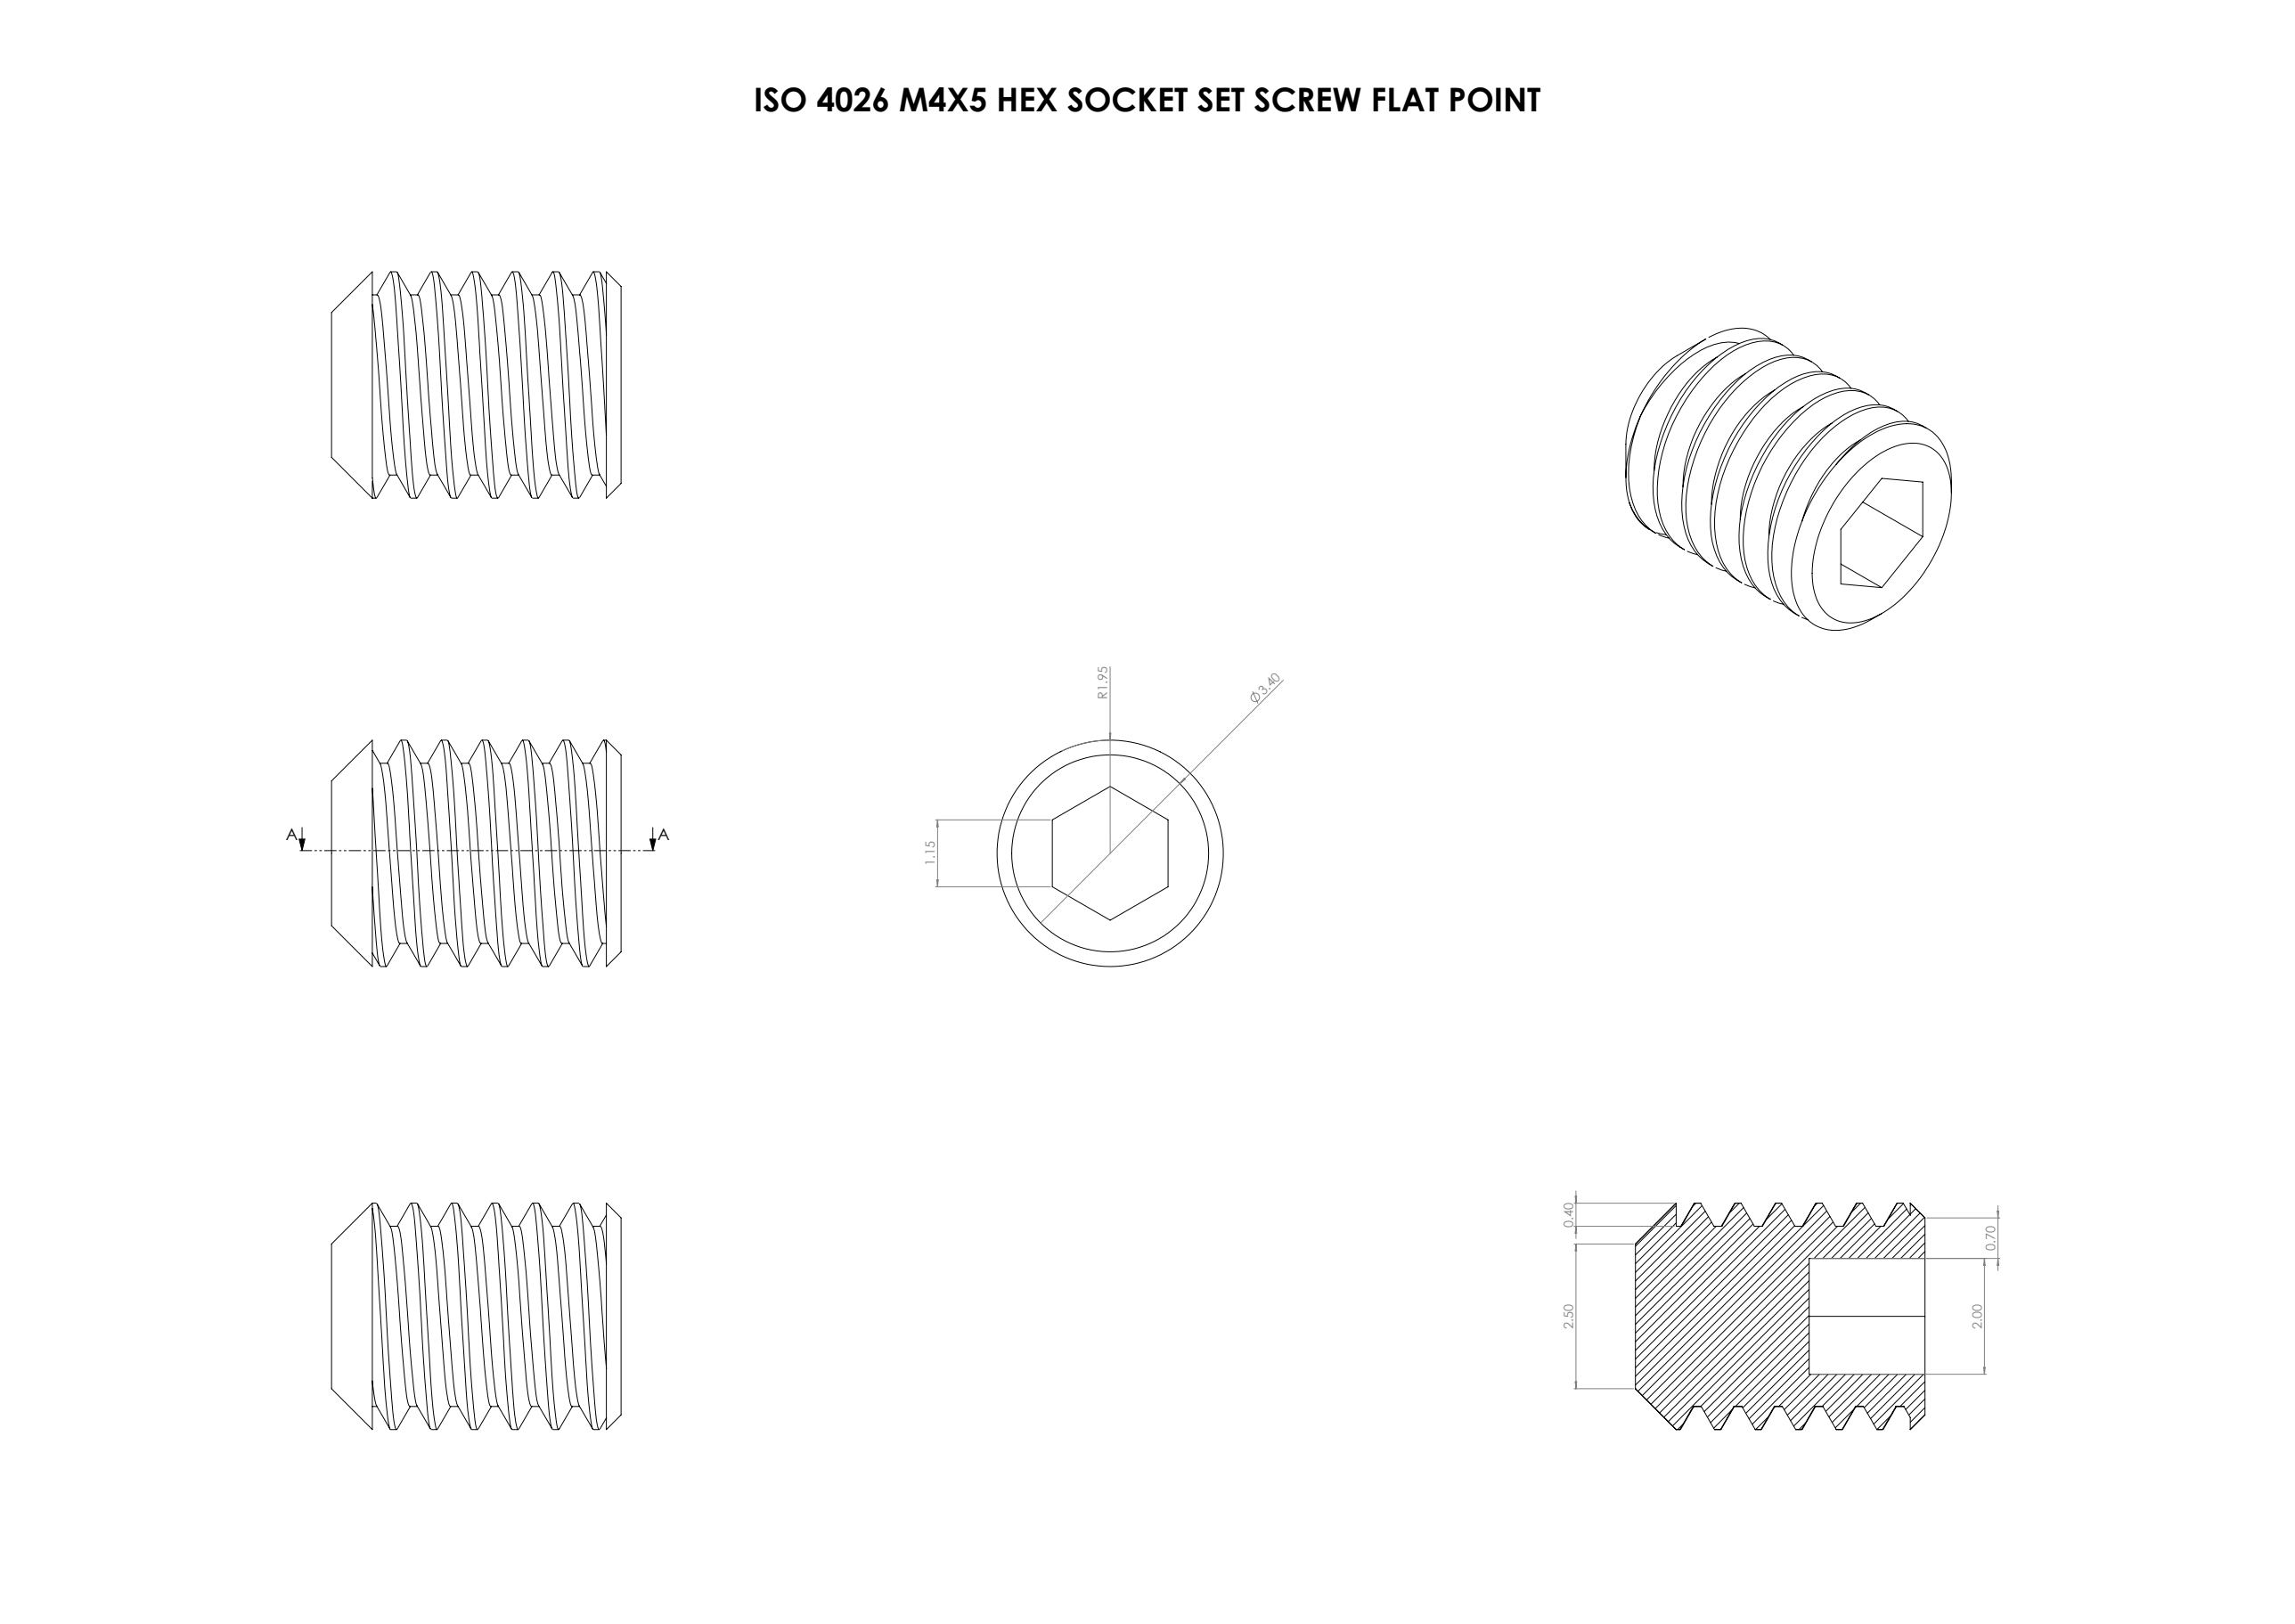
ISO-10303-21;
HEADER;
/* Generated by software containing ST-Developer
 * from STEP Tools, Inc. (www.steptools.com) 
 */

FILE_DESCRIPTION(
/* description */ (''),
/* implementation_level */ '2;1');

FILE_NAME(
/* name */ 
'08_ISO_4026_M4x5_Hex_Socket_Set_Screw_Flat_Point.step',
/* time_stamp */ '2026-10-22T00:21:42-07:00',
/* author */ (''),
/* organization */ (''),
/* preprocessor_version */ 'ST-DEVELOPER v20.2',
/* originating_system */ 'Autodesk Translation Framework v15.15.0.0',
/* authorisation */ '');

FILE_SCHEMA (('AUTOMOTIVE_DESIGN { 1 0 10303 214 3 1 1 }'));
ENDSEC;

DATA;
#10=MECHANICAL_DESIGN_GEOMETRIC_PRESENTATION_REPRESENTATION('',(#212),#31638);
#190=SHAPE_REPRESENTATION_RELATIONSHIP('SRR','None',#31712,#201);
#201=ADVANCED_BREP_SHAPE_REPRESENTATION('',(#223),#31634);
#212=STYLED_ITEM('',(#31837),#223);
#223=MANIFOLD_SOLID_BREP('Set screw',#12487);
#293=CYLINDRICAL_SURFACE('',#13137,0.1954);
#294=CYLINDRICAL_SURFACE('',#13139,0.1954);
#295=CYLINDRICAL_SURFACE('',#13140,0.1954);
#296=CYLINDRICAL_SURFACE('',#13141,0.1954);
#297=CYLINDRICAL_SURFACE('',#13142,0.1954);
#298=CYLINDRICAL_SURFACE('',#13143,0.1954);
#299=CYLINDRICAL_SURFACE('',#13144,0.15555);
#300=CYLINDRICAL_SURFACE('',#13146,0.15555);
#301=CYLINDRICAL_SURFACE('',#13148,0.15555);
#302=CYLINDRICAL_SURFACE('',#13149,0.15555);
#303=CYLINDRICAL_SURFACE('',#13150,0.15555);
#304=CYLINDRICAL_SURFACE('',#13151,0.15555);
#305=CYLINDRICAL_SURFACE('',#13159,0.15555);
#306=CYLINDRICAL_SURFACE('',#13170,0.1954);
#435=CONICAL_SURFACE('',#13169,0.185,0.785398163397445);
#436=CONICAL_SURFACE('',#13172,0.1625,0.785398163397447);
#1015=B_SPLINE_CURVE_WITH_KNOTS('',3,(#25849,#25850,#25851,#25852,#25853,
#25854,#25855,#25856,#25857,#25858),.UNSPECIFIED.,.F.,.F.,(4,3,3,4),(-4.09254174883833,
-3.93292792746001,-2.94969594559501,-2.0651401332781),.UNSPECIFIED.);
#1016=B_SPLINE_CURVE_WITH_KNOTS('',3,(#25861,#25862,#25863,#25864,#25865,
#25866,#25867),.UNSPECIFIED.,.F.,.F.,(4,3,4),(0.,0.983231981865002,1.11419103802958),
 .UNSPECIFIED.);
#1017=B_SPLINE_CURVE_WITH_KNOTS('',3,(#25872,#25873,#25874,#25875,#25876,
#25877,#25878,#25879,#25880,#25881,#25882,#25883,#25884,#25885,#25886,#25887,
#25888,#25889,#25890,#25891,#25892,#25893),.UNSPECIFIED.,.F.,.F.,(4,3,3,
3,3,3,3,4),(-10.3757270560179,-9.83231981865002,-8.84908783678502,-7.86585585492002,
-6.88262387305502,-5.89939189119002,-4.91615990932501,-4.09254174883833),
 .UNSPECIFIED.);
#1018=B_SPLINE_CURVE_WITH_KNOTS('',3,(#25894,#25895,#25896,#25897,#25898,
#25899,#25900,#25901,#25902,#25903,#25904,#25905,#25906,#25907,#25908,#25909,
#25910,#25911,#25912,#25913,#25914,#25915),.UNSPECIFIED.,.F.,.F.,(4,3,3,
3,3,3,3,4),(1.11419103802958,1.96646396373,2.94969594559501,3.93292792746001,
4.91615990932501,5.89939189119001,6.88262387305501,7.39737634520916),
 .UNSPECIFIED.);
#1019=B_SPLINE_CURVE_WITH_KNOTS('',3,(#25920,#25921,#25922,#25923,#25924,
#25925,#25926,#25927,#25928,#25929,#25930,#25931,#25932,#25933,#25934,#25935,
#25936,#25937,#25938,#25939,#25940,#25941),.UNSPECIFIED.,.F.,.F.,(4,3,3,
3,3,3,3,4),(-16.6589123631975,-15.73171170984,-14.748479727975,-13.76524774611,
-12.782015764245,-11.79878378238,-10.815551800515,-10.3757270560179),
 .UNSPECIFIED.);
#1020=B_SPLINE_CURVE_WITH_KNOTS('',3,(#25942,#25943,#25944,#25945,#25946,
#25947,#25948,#25949,#25950,#25951,#25952,#25953,#25954,#25955,#25956,#25957,
#25958,#25959,#25960,#25961,#25962,#25963),.UNSPECIFIED.,.F.,.F.,(4,3,3,
3,3,3,3,4),(7.39737634520916,7.86585585492002,8.84908783678502,9.83231981865002,
10.815551800515,11.79878378238,12.782015764245,13.6805616523888),
 .UNSPECIFIED.);
#1021=B_SPLINE_CURVE_WITH_KNOTS('',3,(#25968,#25969,#25970,#25971,#25972,
#25973,#25974,#25975,#25976,#25977,#25978,#25979,#25980,#25981,#25982,#25983,
#25984,#25985,#25986,#25987,#25988,#25989,#25990,#25991,#25992),
 .UNSPECIFIED.,.F.,.F.,(4,3,3,3,3,3,3,3,4),(-22.9420976703771,-22.6143355828951,
-21.6311036010301,-20.647871619165,-19.6646396373,-18.681407655435,-17.69817567357,
-16.714943691705,-16.6589123631975),.UNSPECIFIED.);
#1022=B_SPLINE_CURVE_WITH_KNOTS('',3,(#25993,#25994,#25995,#25996,#25997,
#25998,#25999,#26000,#26001,#26002,#26003,#26004,#26005,#26006,#26007,#26008,
#26009,#26010,#26011,#26012,#26013,#26014,#26015,#26016,#26017),
 .UNSPECIFIED.,.F.,.F.,(4,3,3,3,3,3,3,3,4),(13.6805616523888,13.76524774611,
14.748479727975,15.73171170984,16.714943691705,17.69817567357,18.681407655435,
19.6646396373,19.9637469595683),.UNSPECIFIED.);
#1023=B_SPLINE_CURVE_WITH_KNOTS('',3,(#26022,#26023,#26024,#26025,#26026,
#26027,#26028,#26029,#26030,#26031,#26032,#26033,#26034,#26035,#26036,#26037,
#26038,#26039,#26040,#26041,#26042,#26043),.UNSPECIFIED.,.F.,.F.,(4,3,3,
3,3,3,3,4),(-29.2252829775567,-28.5137274740851,-27.5304954922201,-26.5472635103551,
-25.5640315284901,-24.5807995466251,-23.5975675647601,-22.9420976703771),
 .UNSPECIFIED.);
#1024=B_SPLINE_CURVE_WITH_KNOTS('',3,(#26044,#26045,#26046,#26047,#26048,
#26049,#26050,#26051,#26052,#26053,#26054,#26055,#26056,#26057,#26058,#26059,
#26060,#26061,#26062,#26063,#26064,#26065),.UNSPECIFIED.,.F.,.F.,(4,3,3,
3,3,3,3,4),(19.9637469595683,20.647871619165,21.63110360103,22.614335582895,
23.59756756476,24.580799546625,25.5640315284901,26.2469322667479),
 .UNSPECIFIED.);
#1025=B_SPLINE_CURVE_WITH_KNOTS('',3,(#26070,#26071,#26072,#26073,#26074,
#26075,#26076,#26077,#26078,#26079,#26080,#26081,#26082,#26083,#26084,#26085,
#26086,#26087,#26088,#26089,#26090,#26091,#26092,#26093,#26094),
 .UNSPECIFIED.,.F.,.F.,(4,3,3,3,3,3,3,3,4),(-35.5084682847363,-35.3963513471401,
-34.4131193652751,-33.4298873834101,-32.4466554015451,-31.4634234196801,
-30.4801914378151,-29.4969594559501,-29.2252829775567),.UNSPECIFIED.);
#1026=B_SPLINE_CURVE_WITH_KNOTS('',3,(#26095,#26096,#26097,#26098,#26099,
#26100,#26101,#26102,#26103,#26104,#26105,#26106,#26107,#26108,#26109,#26110,
#26111,#26112,#26113,#26114,#26115,#26116,#26117,#26118,#26119),
 .UNSPECIFIED.,.F.,.F.,(4,3,3,3,3,3,3,3,4),(26.2469322667479,26.547263510355,
27.5304954922201,28.5137274740851,29.4969594559501,30.4801914378151,31.4634234196801,
32.4466554015451,32.5301175739275),.UNSPECIFIED.);
#1027=B_SPLINE_CURVE_WITH_KNOTS('',3,(#26125,#26126,#26127,#26128),
 .UNSPECIFIED.,.F.,.F.,(4,4),(47.1238898038469,47.8963286785676),
 .UNSPECIFIED.);
#1028=B_SPLINE_CURVE_WITH_KNOTS('',3,(#26134,#26135,#26136,#26137,#26138,
#26139,#26140,#26141,#26142,#26143,#26144),.UNSPECIFIED.,.F.,.F.,(4,1,1,
1,1,1,1,1,4),(40.8407044966673,41.1123809750607,42.0956129569257,43.0788449387907,
44.0620769206557,45.0453089025207,46.0285408843857,47.0117728662507,47.1238898038469),
 .UNSPECIFIED.);
#1029=B_SPLINE_CURVE_WITH_KNOTS('',3,(#26147,#26148,#26149,#26150,#26151,
#26152,#26153,#26154,#26155),.UNSPECIFIED.,.F.,.F.,(4,1,1,1,1,1,4),(40.8407044966673,
41.7404743061498,42.7237062880148,43.7069382698798,44.6901702517448,45.6734022336098,
46.6566342154749),.UNSPECIFIED.);
#1030=B_SPLINE_CURVE_WITH_KNOTS('',3,(#26160,#26161,#26162,#26163,#26164,
#26165,#26166,#26167,#26168,#26169),.UNSPECIFIED.,.F.,.F.,(4,1,1,1,1,1,
1,4),(34.5575191894877,35.2129890838707,36.1962210657357,37.1794530476007,
38.1626850294657,39.1459170113307,40.1291489931957,40.8407044966673),
 .UNSPECIFIED.);
#1031=B_SPLINE_CURVE_WITH_KNOTS('',3,(#26170,#26171,#26172,#26173,#26174,
#26175,#26176,#26177,#26178,#26179,#26180),.UNSPECIFIED.,.F.,.F.,(4,1,1,
1,1,1,1,1,4),(34.5575191894877,34.8578504330948,35.8410824149598,36.8243143968248,
37.8075463786898,38.7907783605548,39.7740103424198,40.7572423242848,40.8407044966673),
 .UNSPECIFIED.);
#1032=B_SPLINE_CURVE_WITH_KNOTS('',3,(#26185,#26186,#26187,#26188,#26189,
#26190,#26191,#26192,#26193,#26194,#26195),.UNSPECIFIED.,.F.,.F.,(4,1,1,
1,1,1,1,1,4),(28.2743338823081,28.3303652108157,29.3135971926807,30.2968291745457,
31.2800611564107,32.2632931382757,33.2465251201407,34.2297571020057,34.5575191894877),
 .UNSPECIFIED.);
#1033=B_SPLINE_CURVE_WITH_KNOTS('',3,(#26196,#26197,#26198,#26199,#26200,
#26201,#26202,#26203,#26204,#26205),.UNSPECIFIED.,.F.,.F.,(4,1,1,1,1,1,
1,4),(28.2743338823081,28.9584585419048,29.9416905237698,30.9249225056348,
31.9081544874998,32.8913864693648,33.8746184512298,34.5575191894877),
 .UNSPECIFIED.);
#1034=B_SPLINE_CURVE_WITH_KNOTS('',3,(#26210,#26211,#26212,#26213,#26214,
#26215,#26216,#26217,#26218,#26219),.UNSPECIFIED.,.F.,.F.,(4,1,1,1,1,1,
1,4),(21.9911485751285,22.4309733196257,23.4142053014907,24.3974372833557,
25.3806692652207,26.3639012470857,27.3471332289507,28.2743338823081),
 .UNSPECIFIED.);
#1035=B_SPLINE_CURVE_WITH_KNOTS('',3,(#26220,#26221,#26222,#26223,#26224,
#26225,#26226,#26227,#26228,#26229,#26230),.UNSPECIFIED.,.F.,.F.,(4,1,1,
1,1,1,1,1,4),(21.9911485751285,22.0758346688498,23.0590666507148,24.0422986325798,
25.0255306144448,26.0087625963098,26.9919945781748,27.9752265600398,28.2743338823081),
 .UNSPECIFIED.);
#1036=B_SPLINE_CURVE_WITH_KNOTS('',3,(#26235,#26236,#26237,#26238,#26239,
#26240,#26241,#26242,#26243,#26244),.UNSPECIFIED.,.F.,.F.,(4,1,1,1,1,1,
1,4),(15.707963267949,16.5315814284356,17.5148134103006,18.4980453921656,
19.4812773740306,20.4645093558957,21.4477413377607,21.9911485751285),
 .UNSPECIFIED.);
#1037=B_SPLINE_CURVE_WITH_KNOTS('',3,(#26245,#26246,#26247,#26248,#26249,
#26250,#26251,#26252,#26253,#26254),.UNSPECIFIED.,.F.,.F.,(4,1,1,1,1,1,
1,4),(15.707963267949,16.1764427776598,17.1596747595248,18.1429067413898,
19.1261387232548,20.1093707051198,21.0926026869848,21.9911485751285),
 .UNSPECIFIED.);
#1038=B_SPLINE_CURVE_WITH_KNOTS('',3,(#26257,#26258,#26259,#26260,#26261,
#26262,#26263,#26264,#26265,#26266,#26267,#26268,#26269,#26270,#26271,#26272,
#26273,#26274,#26275,#26276,#26277,#26278,#26279,#26280,#26281,#26282,#26283,
#26284,#26285,#26286,#26287,#26288,#26289,#26290,#26291,#26292,#26293,#26294,
#26295,#26296,#26297,#26298,#26299,#26300,#26301,#26302,#26303,#26304,#26305,
#26306,#26307,#26308),.UNSPECIFIED.,.F.,.F.,(4,3,3,3,3,3,3,3,3,3,3,3,3,
3,3,3,3,4),(-0.366397579005844,-0.350753953906653,-0.330463017686532,-0.315435531128199,
-0.287643881494464,-0.272924732924834,-0.237814891323476,-0.221795460451242,
-0.207726041133023,-0.184571159408416,-0.160894855415823,-0.147419681563097,
-0.13576580392061,-0.101824352940458,-0.0769585672558313,-0.0671142413070353,
-0.0286195295740189,0.),.UNSPECIFIED.);
#1039=B_SPLINE_CURVE_WITH_KNOTS('',3,(#26313,#26314,#26315,#26316,#26317,
#26318,#26319,#26320,#26321,#26322,#26323,#26324,#26325,#26326,#26327,#26328,
#26329,#26330,#26331,#26332,#26333,#26334,#26335,#26336,#26337,#26338,#26339,
#26340,#26341,#26342,#26343,#26344,#26345,#26346,#26347,#26348,#26349,#26350,
#26351,#26352,#26353,#26354,#26355,#26356,#26357,#26358,#26359,#26360,#26361,
#26362,#26363,#26364,#26365,#26366,#26367),.UNSPECIFIED.,.F.,.F.,(4,3,3,
3,3,3,3,3,3,3,3,3,3,3,3,3,3,3,4),(-0.364629307890667,-0.345405509511423,
-0.316109491299348,-0.303964239439482,-0.281709554317525,-0.264921543558191,
-0.252375276770721,-0.215944087132777,-0.198753901855764,-0.18596810420685,
-0.163689794923203,-0.143278793185558,-0.127728424538677,-0.117434610457182,
-0.0880759578428862,-0.0702652452140735,-0.0601818930641948,-0.0277041096514565,
0.),.UNSPECIFIED.);
#1040=B_SPLINE_CURVE_WITH_KNOTS('',3,(#26536,#26537,#26538,#26539,#26540,
#26541,#26542,#26543,#26544,#26545,#26546,#26547,#26548),.UNSPECIFIED.,
 .F.,.F.,(4,3,3,3,4),(32.5301175739275,33.4298873834101,34.4131193652751,
35.3963513471401,36.280907159457),.UNSPECIFIED.);
#1041=B_SPLINE_CURVE_WITH_KNOTS('',3,(#26550,#26551,#26552,#26553,#26554,
#26555,#26556,#26557,#26558,#26559,#26560,#26561,#26562,#26563,#26564,#26565,
#26566,#26567,#26568,#26569,#26570,#26571,#26572,#26573,#26574,#26575,#26576,
#26577,#26578,#26579,#26580,#26581,#26582,#26583,#26584,#26585,#26586,#26587,
#26588,#26589,#26590,#26591,#26592,#26593,#26594,#26595,#26596,#26597,#26598,
#26599,#26600,#26601),.UNSPECIFIED.,.F.,.F.,(4,3,3,3,3,3,3,3,3,3,3,3,3,
3,3,3,3,4),(-0.366397579005851,-0.350753953906661,-0.330463024735024,-0.315435543259483,
-0.287644877982493,-0.272925011059114,-0.237815179368718,-0.221795848896316,
-0.207726060922694,-0.184571159408424,-0.160894850055595,-0.147419600331868,
-0.135765787605129,-0.101824340703847,-0.0769585196865098,-0.0671141722159687,
-0.0286194368321035,0.),.UNSPECIFIED.);
#1042=B_SPLINE_CURVE_WITH_KNOTS('',3,(#26602,#26603,#26604,#26605,#26606,
#26607,#26608,#26609,#26610),.UNSPECIFIED.,.F.,.F.,(4,1,1,1,1,1,4),(10.3757270560179,
11.2602828683348,12.2435148501998,13.2267468320648,14.2099788139298,15.1932107957948,
15.707963267949),.UNSPECIFIED.);
#1043=B_SPLINE_CURVE_WITH_KNOTS('',3,(#26616,#26617,#26618,#26619,#26620,
#26621,#26622,#26623,#26624,#26625,#26626,#26627,#26628,#26629,#26630,#26631,
#26632,#26633,#26634,#26635,#26636,#26637,#26638,#26639,#26640,#26641,#26642,
#26643,#26644,#26645,#26646,#26647,#26648,#26649,#26650,#26651,#26652,#26653,
#26654,#26655,#26656,#26657,#26658,#26659,#26660,#26661,#26662,#26663,#26664,
#26665,#26666,#26667,#26668,#26669,#26670),.UNSPECIFIED.,.F.,.F.,(4,3,3,
3,3,3,3,3,3,3,3,3,3,3,3,3,3,3,4),(-0.364629307890684,-0.345405509511438,
-0.316109466616483,-0.303964180518109,-0.28170938055002,-0.264921036000774,
-0.252375151029453,-0.215943930999405,-0.198753706254068,-0.185968021399695,
-0.163689794923211,-0.143278681804942,-0.127728193637607,-0.117434275921994,
-0.0880757069414953,-0.070264744543059,-0.0601814248546799,-0.0277037327266843,
0.),.UNSPECIFIED.);
#1044=B_SPLINE_CURVE_WITH_KNOTS('',3,(#26673,#26674,#26675,#26676,#26677,
#26678,#26679,#26680),.UNSPECIFIED.,.F.,.F.,(4,1,1,1,1,4),(11.6154215191106,
12.5986535009756,13.5818854828406,14.5651174647056,15.5483494465706,15.707963267949),
 .UNSPECIFIED.);
#1045=B_SPLINE_CURVE_WITH_KNOTS('',3,(#26849,#26850,#26851,#26852,#26853,
#26854,#26855,#26856,#26857,#26858),.UNSPECIFIED.,.F.,.F.,(4,3,3,4),(-38.3460472927351,
-37.3628153108701,-36.3795833290051,-35.5084682847363),.UNSPECIFIED.);
#1330=B_SPLINE_SURFACE_WITH_KNOTS('',3,3,((#26368,#26369,#26370,#26371,
#26372,#26373,#26374,#26375,#26376,#26377,#26378,#26379,#26380,#26381,#26382,
#26383,#26384,#26385,#26386,#26387,#26388,#26389,#26390,#26391,#26392,#26393,
#26394,#26395,#26396,#26397,#26398,#26399,#26400,#26401,#26402,#26403,#26404,
#26405,#26406,#26407,#26408,#26409),(#26410,#26411,#26412,#26413,#26414,
#26415,#26416,#26417,#26418,#26419,#26420,#26421,#26422,#26423,#26424,#26425,
#26426,#26427,#26428,#26429,#26430,#26431,#26432,#26433,#26434,#26435,#26436,
#26437,#26438,#26439,#26440,#26441,#26442,#26443,#26444,#26445,#26446,#26447,
#26448,#26449,#26450,#26451),(#26452,#26453,#26454,#26455,#26456,#26457,
#26458,#26459,#26460,#26461,#26462,#26463,#26464,#26465,#26466,#26467,#26468,
#26469,#26470,#26471,#26472,#26473,#26474,#26475,#26476,#26477,#26478,#26479,
#26480,#26481,#26482,#26483,#26484,#26485,#26486,#26487,#26488,#26489,#26490,
#26491,#26492,#26493),(#26494,#26495,#26496,#26497,#26498,#26499,#26500,
#26501,#26502,#26503,#26504,#26505,#26506,#26507,#26508,#26509,#26510,#26511,
#26512,#26513,#26514,#26515,#26516,#26517,#26518,#26519,#26520,#26521,#26522,
#26523,#26524,#26525,#26526,#26527,#26528,#26529,#26530,#26531,#26532,#26533,
#26534,#26535)),.UNSPECIFIED.,.F.,.F.,.F.,(4,4),(4,1,1,1,1,1,1,1,1,1,1,
1,1,1,1,1,1,1,1,1,1,1,1,1,1,1,1,1,1,1,1,1,1,1,1,1,1,1,1,4),(0.,0.0460148164544131),
(8.31058692273978,9.29381890460478,10.2770508864698,11.2602828683348,12.2435148501998,
13.2267468320648,14.2099788139298,15.1932107957948,16.1764427776598,17.1596747595248,
18.1429067413898,19.1261387232548,20.1093707051198,21.0926026869848,22.0758346688498,
23.0590666507148,24.0422986325798,25.0255306144448,26.0087625963098,26.9919945781748,
27.9752265600398,28.9584585419048,29.9416905237698,30.9249225056348,31.9081544874998,
32.8913864693648,33.8746184512298,34.8578504330948,35.8410824149598,36.8243143968248,
37.8075463786898,38.7907783605548,39.7740103424198,40.7572423242848,41.7404743061498,
42.7237062880148,43.7069382698798,44.6901702517448,45.6734022336098,46.6566342154749),
 .UNSPECIFIED.);
#1331=B_SPLINE_SURFACE_WITH_KNOTS('',3,3,((#26681,#26682,#26683,#26684,
#26685,#26686,#26687,#26688,#26689,#26690,#26691,#26692,#26693,#26694,#26695,
#26696,#26697,#26698,#26699,#26700,#26701,#26702,#26703,#26704,#26705,#26706,
#26707,#26708,#26709,#26710,#26711,#26712,#26713,#26714,#26715,#26716,#26717,
#26718,#26719,#26720,#26721,#26722),(#26723,#26724,#26725,#26726,#26727,
#26728,#26729,#26730,#26731,#26732,#26733,#26734,#26735,#26736,#26737,#26738,
#26739,#26740,#26741,#26742,#26743,#26744,#26745,#26746,#26747,#26748,#26749,
#26750,#26751,#26752,#26753,#26754,#26755,#26756,#26757,#26758,#26759,#26760,
#26761,#26762,#26763,#26764),(#26765,#26766,#26767,#26768,#26769,#26770,
#26771,#26772,#26773,#26774,#26775,#26776,#26777,#26778,#26779,#26780,#26781,
#26782,#26783,#26784,#26785,#26786,#26787,#26788,#26789,#26790,#26791,#26792,
#26793,#26794,#26795,#26796,#26797,#26798,#26799,#26800,#26801,#26802,#26803,
#26804,#26805,#26806),(#26807,#26808,#26809,#26810,#26811,#26812,#26813,
#26814,#26815,#26816,#26817,#26818,#26819,#26820,#26821,#26822,#26823,#26824,
#26825,#26826,#26827,#26828,#26829,#26830,#26831,#26832,#26833,#26834,#26835,
#26836,#26837,#26838,#26839,#26840,#26841,#26842,#26843,#26844,#26845,#26846,
#26847,#26848)),.UNSPECIFIED.,.F.,.F.,.F.,(4,4),(4,1,1,1,1,1,1,1,1,1,1,
1,1,1,1,1,1,1,1,1,1,1,1,1,1,1,1,1,1,1,1,1,1,1,1,1,1,1,1,4),(0.,0.0460148164544132),
(11.6154215191106,12.5986535009756,13.5818854828406,14.5651174647056,15.5483494465706,
16.5315814284356,17.5148134103006,18.4980453921656,19.4812773740306,20.4645093558957,
21.4477413377607,22.4309733196257,23.4142053014907,24.3974372833557,25.3806692652207,
26.3639012470857,27.3471332289507,28.3303652108157,29.3135971926807,30.2968291745457,
31.2800611564107,32.2632931382757,33.2465251201407,34.2297571020057,35.2129890838707,
36.1962210657357,37.1794530476007,38.1626850294657,39.1459170113307,40.1291489931957,
41.1123809750607,42.0956129569257,43.0788449387907,44.0620769206557,45.0453089025207,
46.0285408843857,47.0117728662507,47.9950048481157,48.9782368299807,49.9614688118457),
 .UNSPECIFIED.);
#1396=FACE_BOUND('',#2997,.T.);
#1657=CIRCLE('',#13138,0.1954);
#1658=CIRCLE('',#13145,0.15555);
#1659=CIRCLE('',#13147,0.15555);
#1660=CIRCLE('',#13153,0.1954);
#1661=CIRCLE('',#13154,0.1954);
#1662=CIRCLE('',#13156,0.1954);
#1663=CIRCLE('',#13157,0.1954);
#1664=CIRCLE('',#13158,0.15555);
#1665=CIRCLE('',#13168,0.17);
#1666=CIRCLE('',#13171,0.1954);
#1667=CIRCLE('',#13173,0.125);
#2222=FACE_OUTER_BOUND('',#2972,.T.);
#2223=FACE_OUTER_BOUND('',#2973,.T.);
#2224=FACE_OUTER_BOUND('',#2974,.T.);
#2225=FACE_OUTER_BOUND('',#2975,.T.);
#2226=FACE_OUTER_BOUND('',#2976,.T.);
#2227=FACE_OUTER_BOUND('',#2977,.T.);
#2228=FACE_OUTER_BOUND('',#2978,.T.);
#2229=FACE_OUTER_BOUND('',#2979,.T.);
#2230=FACE_OUTER_BOUND('',#2980,.T.);
#2231=FACE_OUTER_BOUND('',#2981,.T.);
#2232=FACE_OUTER_BOUND('',#2982,.T.);
#2233=FACE_OUTER_BOUND('',#2983,.T.);
#2234=FACE_OUTER_BOUND('',#2984,.T.);
#2235=FACE_OUTER_BOUND('',#2985,.T.);
#2236=FACE_OUTER_BOUND('',#2986,.T.);
#2237=FACE_OUTER_BOUND('',#2987,.T.);
#2238=FACE_OUTER_BOUND('',#2988,.T.);
#2239=FACE_OUTER_BOUND('',#2989,.T.);
#2240=FACE_OUTER_BOUND('',#2990,.T.);
#2241=FACE_OUTER_BOUND('',#2991,.T.);
#2242=FACE_OUTER_BOUND('',#2992,.T.);
#2243=FACE_OUTER_BOUND('',#2993,.T.);
#2244=FACE_OUTER_BOUND('',#2994,.T.);
#2245=FACE_OUTER_BOUND('',#2995,.T.);
#2246=FACE_OUTER_BOUND('',#2996,.T.);
#2247=FACE_OUTER_BOUND('',#2998,.T.);
#2248=FACE_OUTER_BOUND('',#2999,.T.);
#2249=FACE_OUTER_BOUND('',#3000,.T.);
#2250=FACE_OUTER_BOUND('',#3001,.T.);
#2972=EDGE_LOOP('',(#10017,#10018,#10019,#10020));
#2973=EDGE_LOOP('',(#10021,#10022,#10023,#10024));
#2974=EDGE_LOOP('',(#10025,#10026,#10027,#10028));
#2975=EDGE_LOOP('',(#10029,#10030,#10031,#10032));
#2976=EDGE_LOOP('',(#10033,#10034,#10035,#10036));
#2977=EDGE_LOOP('',(#10037,#10038,#10039,#10040));
#2978=EDGE_LOOP('',(#10041,#10042,#10043));
#2979=EDGE_LOOP('',(#10044,#10045,#10046,#10047,#10048));
#2980=EDGE_LOOP('',(#10049,#10050,#10051,#10052));
#2981=EDGE_LOOP('',(#10053,#10054,#10055,#10056));
#2982=EDGE_LOOP('',(#10057,#10058,#10059,#10060));
#2983=EDGE_LOOP('',(#10061,#10062,#10063,#10064));
#2984=EDGE_LOOP('',(#10065,#10066,#10067,#10068,#10069,#10070));
#2985=EDGE_LOOP('',(#10071,#10072,#10073,#10074,#10075,#10076,#10077,#10078,
#10079,#10080,#10081,#10082,#10083,#10084,#10085));
#2986=EDGE_LOOP('',(#10086,#10087,#10088,#10089,#10090));
#2987=EDGE_LOOP('',(#10091,#10092,#10093,#10094));
#2988=EDGE_LOOP('',(#10095,#10096,#10097,#10098,#10099,#10100,#10101,#10102,
#10103,#10104,#10105,#10106,#10107,#10108,#10109,#10110));
#2989=EDGE_LOOP('',(#10111,#10112,#10113,#10114));
#2990=EDGE_LOOP('',(#10115,#10116,#10117,#10118));
#2991=EDGE_LOOP('',(#10119,#10120,#10121,#10122));
#2992=EDGE_LOOP('',(#10123,#10124,#10125,#10126));
#2993=EDGE_LOOP('',(#10127,#10128,#10129,#10130));
#2994=EDGE_LOOP('',(#10131,#10132,#10133,#10134));
#2995=EDGE_LOOP('',(#10135,#10136,#10137,#10138,#10139,#10140));
#2996=EDGE_LOOP('',(#10141));
#2997=EDGE_LOOP('',(#10142,#10143,#10144,#10145,#10146,#10147));
#2998=EDGE_LOOP('',(#10148,#10149,#10150,#10151,#10152,#10153));
#2999=EDGE_LOOP('',(#10154,#10155,#10156,#10157));
#3000=EDGE_LOOP('',(#10158,#10159,#10160,#10161,#10162,#10163));
#3001=EDGE_LOOP('',(#10164));
#3590=LINE('',#25847,#4295);
#3591=LINE('',#25871,#4296);
#3592=LINE('',#25919,#4297);
#3593=LINE('',#25967,#4298);
#3594=LINE('',#26021,#4299);
#3595=LINE('',#26069,#4300);
#3596=LINE('',#26123,#4301);
#3597=LINE('',#26133,#4302);
#3598=LINE('',#26159,#4303);
#3599=LINE('',#26184,#4304);
#3600=LINE('',#26209,#4305);
#3601=LINE('',#26234,#4306);
#3602=LINE('',#26862,#4307);
#3603=LINE('',#26864,#4308);
#3604=LINE('',#26866,#4309);
#3605=LINE('',#26867,#4310);
#3606=LINE('',#26870,#4311);
#3607=LINE('',#26872,#4312);
#3608=LINE('',#26873,#4313);
#3609=LINE('',#26876,#4314);
#3610=LINE('',#26878,#4315);
#3611=LINE('',#26879,#4316);
#3612=LINE('',#26882,#4317);
#3613=LINE('',#26884,#4318);
#3614=LINE('',#26885,#4319);
#3615=LINE('',#26888,#4320);
#3616=LINE('',#26890,#4321);
#3617=LINE('',#26891,#4322);
#3618=LINE('',#26893,#4323);
#3619=LINE('',#26894,#4324);
#3620=LINE('',#26900,#4325);
#3621=LINE('',#26906,#4326);
#4295=VECTOR('',#14988,0.2);
#4296=VECTOR('',#14993,0.2);
#4297=VECTOR('',#14996,0.2);
#4298=VECTOR('',#14999,0.2);
#4299=VECTOR('',#15002,0.2);
#4300=VECTOR('',#15005,0.2);
#4301=VECTOR('',#15008,0.15555);
#4302=VECTOR('',#15013,0.15555);
#4303=VECTOR('',#15018,0.15555);
#4304=VECTOR('',#15021,0.15555);
#4305=VECTOR('',#15024,0.15555);
#4306=VECTOR('',#15027,0.15555);
#4307=VECTOR('',#15046,1.);
#4308=VECTOR('',#15047,1.);
#4309=VECTOR('',#15048,1.);
#4310=VECTOR('',#15049,1.);
#4311=VECTOR('',#15052,1.);
#4312=VECTOR('',#15053,1.);
#4313=VECTOR('',#15054,1.);
#4314=VECTOR('',#15057,1.);
#4315=VECTOR('',#15058,1.);
#4316=VECTOR('',#15059,1.);
#4317=VECTOR('',#15062,1.);
#4318=VECTOR('',#15063,1.);
#4319=VECTOR('',#15064,1.);
#4320=VECTOR('',#15067,1.);
#4321=VECTOR('',#15068,1.);
#4322=VECTOR('',#15069,1.);
#4323=VECTOR('',#15072,1.);
#4324=VECTOR('',#15073,1.);
#4325=VECTOR('',#15082,0.185);
#4326=VECTOR('',#15091,0.1625);
#5433=VERTEX_POINT('',#25845);
#5434=VERTEX_POINT('',#25846);
#5435=VERTEX_POINT('',#25848);
#5436=VERTEX_POINT('',#25859);
#5437=VERTEX_POINT('',#25869);
#5438=VERTEX_POINT('',#25870);
#5439=VERTEX_POINT('',#25917);
#5440=VERTEX_POINT('',#25918);
#5441=VERTEX_POINT('',#25965);
#5442=VERTEX_POINT('',#25966);
#5443=VERTEX_POINT('',#26019);
#5444=VERTEX_POINT('',#26020);
#5445=VERTEX_POINT('',#26067);
#5446=VERTEX_POINT('',#26068);
#5447=VERTEX_POINT('',#26121);
#5448=VERTEX_POINT('',#26122);
#5449=VERTEX_POINT('',#26124);
#5450=VERTEX_POINT('',#26131);
#5451=VERTEX_POINT('',#26132);
#5452=VERTEX_POINT('',#26145);
#5453=VERTEX_POINT('',#26157);
#5454=VERTEX_POINT('',#26158);
#5455=VERTEX_POINT('',#26182);
#5456=VERTEX_POINT('',#26183);
#5457=VERTEX_POINT('',#26207);
#5458=VERTEX_POINT('',#26208);
#5459=VERTEX_POINT('',#26232);
#5460=VERTEX_POINT('',#26233);
#5461=VERTEX_POINT('',#26256);
#5462=VERTEX_POINT('',#26309);
#5463=VERTEX_POINT('',#26311);
#5464=VERTEX_POINT('',#26549);
#5465=VERTEX_POINT('',#26612);
#5466=VERTEX_POINT('',#26615);
#5467=VERTEX_POINT('',#26860);
#5468=VERTEX_POINT('',#26861);
#5469=VERTEX_POINT('',#26863);
#5470=VERTEX_POINT('',#26865);
#5471=VERTEX_POINT('',#26869);
#5472=VERTEX_POINT('',#26871);
#5473=VERTEX_POINT('',#26875);
#5474=VERTEX_POINT('',#26877);
#5475=VERTEX_POINT('',#26881);
#5476=VERTEX_POINT('',#26883);
#5477=VERTEX_POINT('',#26887);
#5478=VERTEX_POINT('',#26889);
#5479=VERTEX_POINT('',#26897);
#5480=VERTEX_POINT('',#26904);
#7020=EDGE_CURVE('',#5433,#5434,#3590,.T.);
#7021=EDGE_CURVE('',#5433,#5435,#1015,.T.);
#7022=EDGE_CURVE('',#5435,#5436,#1657,.T.);
#7023=EDGE_CURVE('',#5436,#5434,#1016,.T.);
#7024=EDGE_CURVE('',#5437,#5438,#3591,.T.);
#7025=EDGE_CURVE('',#5437,#5433,#1017,.T.);
#7026=EDGE_CURVE('',#5434,#5438,#1018,.T.);
#7027=EDGE_CURVE('',#5439,#5440,#3592,.T.);
#7028=EDGE_CURVE('',#5439,#5437,#1019,.T.);
#7029=EDGE_CURVE('',#5438,#5440,#1020,.T.);
#7030=EDGE_CURVE('',#5441,#5442,#3593,.T.);
#7031=EDGE_CURVE('',#5441,#5439,#1021,.T.);
#7032=EDGE_CURVE('',#5440,#5442,#1022,.T.);
#7033=EDGE_CURVE('',#5443,#5444,#3594,.T.);
#7034=EDGE_CURVE('',#5443,#5441,#1023,.T.);
#7035=EDGE_CURVE('',#5442,#5444,#1024,.T.);
#7036=EDGE_CURVE('',#5445,#5446,#3595,.T.);
#7037=EDGE_CURVE('',#5445,#5443,#1025,.T.);
#7038=EDGE_CURVE('',#5444,#5446,#1026,.T.);
#7039=EDGE_CURVE('',#5447,#5448,#3596,.T.);
#7040=EDGE_CURVE('',#5447,#5449,#1027,.T.);
#7041=EDGE_CURVE('',#5448,#5449,#1658,.T.);
#7042=EDGE_CURVE('',#5450,#5451,#3597,.T.);
#7043=EDGE_CURVE('',#5450,#5447,#1028,.T.);
#7044=EDGE_CURVE('',#5452,#5448,#1659,.T.);
#7045=EDGE_CURVE('',#5451,#5452,#1029,.T.);
#7046=EDGE_CURVE('',#5453,#5454,#3598,.T.);
#7047=EDGE_CURVE('',#5453,#5450,#1030,.T.);
#7048=EDGE_CURVE('',#5454,#5451,#1031,.T.);
#7049=EDGE_CURVE('',#5455,#5456,#3599,.T.);
#7050=EDGE_CURVE('',#5455,#5453,#1032,.T.);
#7051=EDGE_CURVE('',#5456,#5454,#1033,.T.);
#7052=EDGE_CURVE('',#5457,#5458,#3600,.T.);
#7053=EDGE_CURVE('',#5457,#5455,#1034,.T.);
#7054=EDGE_CURVE('',#5458,#5456,#1035,.T.);
#7055=EDGE_CURVE('',#5459,#5460,#3601,.T.);
#7056=EDGE_CURVE('',#5459,#5457,#1036,.T.);
#7057=EDGE_CURVE('',#5460,#5458,#1037,.T.);
#7058=EDGE_CURVE('',#5449,#5461,#1038,.T.);
#7059=EDGE_CURVE('',#5462,#5461,#1660,.F.);
#7060=EDGE_CURVE('',#5463,#5462,#1661,.F.);
#7061=EDGE_CURVE('',#5463,#5452,#1039,.T.);
#7062=EDGE_CURVE('',#5446,#5463,#1040,.T.);
#7063=EDGE_CURVE('',#5464,#5436,#1041,.T.);
#7064=EDGE_CURVE('',#5464,#5460,#1042,.T.);
#7065=EDGE_CURVE('',#5436,#5465,#1662,.T.);
#7066=EDGE_CURVE('',#5465,#5435,#1663,.T.);
#7067=EDGE_CURVE('',#5435,#5466,#1043,.T.);
#7068=EDGE_CURVE('',#5466,#5464,#1664,.T.);
#7069=EDGE_CURVE('',#5466,#5459,#1044,.T.);
#7070=EDGE_CURVE('',#5461,#5445,#1045,.T.);
#7071=EDGE_CURVE('',#5467,#5468,#3602,.T.);
#7072=EDGE_CURVE('',#5467,#5469,#3603,.T.);
#7073=EDGE_CURVE('',#5469,#5470,#3604,.T.);
#7074=EDGE_CURVE('',#5468,#5470,#3605,.T.);
#7075=EDGE_CURVE('',#5471,#5467,#3606,.T.);
#7076=EDGE_CURVE('',#5471,#5472,#3607,.T.);
#7077=EDGE_CURVE('',#5472,#5469,#3608,.T.);
#7078=EDGE_CURVE('',#5473,#5471,#3609,.T.);
#7079=EDGE_CURVE('',#5473,#5474,#3610,.T.);
#7080=EDGE_CURVE('',#5474,#5472,#3611,.T.);
#7081=EDGE_CURVE('',#5475,#5473,#3612,.T.);
#7082=EDGE_CURVE('',#5475,#5476,#3613,.T.);
#7083=EDGE_CURVE('',#5476,#5474,#3614,.T.);
#7084=EDGE_CURVE('',#5477,#5475,#3615,.T.);
#7085=EDGE_CURVE('',#5477,#5478,#3616,.T.);
#7086=EDGE_CURVE('',#5478,#5476,#3617,.T.);
#7087=EDGE_CURVE('',#5468,#5477,#3618,.T.);
#7088=EDGE_CURVE('',#5470,#5478,#3619,.T.);
#7089=EDGE_CURVE('',#5479,#5479,#1665,.T.);
#7090=EDGE_CURVE('',#5465,#5479,#3620,.T.);
#7091=EDGE_CURVE('',#5461,#5463,#1666,.F.);
#7092=EDGE_CURVE('',#5480,#5480,#1667,.T.);
#7093=EDGE_CURVE('',#5480,#5462,#3621,.T.);
#10017=ORIENTED_EDGE('',*,*,#7020,.F.);
#10018=ORIENTED_EDGE('',*,*,#7021,.T.);
#10019=ORIENTED_EDGE('',*,*,#7022,.T.);
#10020=ORIENTED_EDGE('',*,*,#7023,.T.);
#10021=ORIENTED_EDGE('',*,*,#7024,.F.);
#10022=ORIENTED_EDGE('',*,*,#7025,.T.);
#10023=ORIENTED_EDGE('',*,*,#7020,.T.);
#10024=ORIENTED_EDGE('',*,*,#7026,.T.);
#10025=ORIENTED_EDGE('',*,*,#7027,.F.);
#10026=ORIENTED_EDGE('',*,*,#7028,.T.);
#10027=ORIENTED_EDGE('',*,*,#7024,.T.);
#10028=ORIENTED_EDGE('',*,*,#7029,.T.);
#10029=ORIENTED_EDGE('',*,*,#7030,.F.);
#10030=ORIENTED_EDGE('',*,*,#7031,.T.);
#10031=ORIENTED_EDGE('',*,*,#7027,.T.);
#10032=ORIENTED_EDGE('',*,*,#7032,.T.);
#10033=ORIENTED_EDGE('',*,*,#7033,.F.);
#10034=ORIENTED_EDGE('',*,*,#7034,.T.);
#10035=ORIENTED_EDGE('',*,*,#7030,.T.);
#10036=ORIENTED_EDGE('',*,*,#7035,.T.);
#10037=ORIENTED_EDGE('',*,*,#7036,.F.);
#10038=ORIENTED_EDGE('',*,*,#7037,.T.);
#10039=ORIENTED_EDGE('',*,*,#7033,.T.);
#10040=ORIENTED_EDGE('',*,*,#7038,.T.);
#10041=ORIENTED_EDGE('',*,*,#7039,.F.);
#10042=ORIENTED_EDGE('',*,*,#7040,.T.);
#10043=ORIENTED_EDGE('',*,*,#7041,.F.);
#10044=ORIENTED_EDGE('',*,*,#7042,.F.);
#10045=ORIENTED_EDGE('',*,*,#7043,.T.);
#10046=ORIENTED_EDGE('',*,*,#7039,.T.);
#10047=ORIENTED_EDGE('',*,*,#7044,.F.);
#10048=ORIENTED_EDGE('',*,*,#7045,.F.);
#10049=ORIENTED_EDGE('',*,*,#7046,.F.);
#10050=ORIENTED_EDGE('',*,*,#7047,.T.);
#10051=ORIENTED_EDGE('',*,*,#7042,.T.);
#10052=ORIENTED_EDGE('',*,*,#7048,.F.);
#10053=ORIENTED_EDGE('',*,*,#7049,.F.);
#10054=ORIENTED_EDGE('',*,*,#7050,.T.);
#10055=ORIENTED_EDGE('',*,*,#7046,.T.);
#10056=ORIENTED_EDGE('',*,*,#7051,.F.);
#10057=ORIENTED_EDGE('',*,*,#7052,.F.);
#10058=ORIENTED_EDGE('',*,*,#7053,.T.);
#10059=ORIENTED_EDGE('',*,*,#7049,.T.);
#10060=ORIENTED_EDGE('',*,*,#7054,.F.);
#10061=ORIENTED_EDGE('',*,*,#7055,.F.);
#10062=ORIENTED_EDGE('',*,*,#7056,.T.);
#10063=ORIENTED_EDGE('',*,*,#7052,.T.);
#10064=ORIENTED_EDGE('',*,*,#7057,.F.);
#10065=ORIENTED_EDGE('',*,*,#7044,.T.);
#10066=ORIENTED_EDGE('',*,*,#7041,.T.);
#10067=ORIENTED_EDGE('',*,*,#7058,.T.);
#10068=ORIENTED_EDGE('',*,*,#7059,.F.);
#10069=ORIENTED_EDGE('',*,*,#7060,.F.);
#10070=ORIENTED_EDGE('',*,*,#7061,.T.);
#10071=ORIENTED_EDGE('',*,*,#7061,.F.);
#10072=ORIENTED_EDGE('',*,*,#7062,.F.);
#10073=ORIENTED_EDGE('',*,*,#7038,.F.);
#10074=ORIENTED_EDGE('',*,*,#7035,.F.);
#10075=ORIENTED_EDGE('',*,*,#7032,.F.);
#10076=ORIENTED_EDGE('',*,*,#7029,.F.);
#10077=ORIENTED_EDGE('',*,*,#7026,.F.);
#10078=ORIENTED_EDGE('',*,*,#7023,.F.);
#10079=ORIENTED_EDGE('',*,*,#7063,.F.);
#10080=ORIENTED_EDGE('',*,*,#7064,.T.);
#10081=ORIENTED_EDGE('',*,*,#7057,.T.);
#10082=ORIENTED_EDGE('',*,*,#7054,.T.);
#10083=ORIENTED_EDGE('',*,*,#7051,.T.);
#10084=ORIENTED_EDGE('',*,*,#7048,.T.);
#10085=ORIENTED_EDGE('',*,*,#7045,.T.);
#10086=ORIENTED_EDGE('',*,*,#7065,.T.);
#10087=ORIENTED_EDGE('',*,*,#7066,.T.);
#10088=ORIENTED_EDGE('',*,*,#7067,.T.);
#10089=ORIENTED_EDGE('',*,*,#7068,.T.);
#10090=ORIENTED_EDGE('',*,*,#7063,.T.);
#10091=ORIENTED_EDGE('',*,*,#7055,.T.);
#10092=ORIENTED_EDGE('',*,*,#7064,.F.);
#10093=ORIENTED_EDGE('',*,*,#7068,.F.);
#10094=ORIENTED_EDGE('',*,*,#7069,.T.);
#10095=ORIENTED_EDGE('',*,*,#7058,.F.);
#10096=ORIENTED_EDGE('',*,*,#7040,.F.);
#10097=ORIENTED_EDGE('',*,*,#7043,.F.);
#10098=ORIENTED_EDGE('',*,*,#7047,.F.);
#10099=ORIENTED_EDGE('',*,*,#7050,.F.);
#10100=ORIENTED_EDGE('',*,*,#7053,.F.);
#10101=ORIENTED_EDGE('',*,*,#7056,.F.);
#10102=ORIENTED_EDGE('',*,*,#7069,.F.);
#10103=ORIENTED_EDGE('',*,*,#7067,.F.);
#10104=ORIENTED_EDGE('',*,*,#7021,.F.);
#10105=ORIENTED_EDGE('',*,*,#7025,.F.);
#10106=ORIENTED_EDGE('',*,*,#7028,.F.);
#10107=ORIENTED_EDGE('',*,*,#7031,.F.);
#10108=ORIENTED_EDGE('',*,*,#7034,.F.);
#10109=ORIENTED_EDGE('',*,*,#7037,.F.);
#10110=ORIENTED_EDGE('',*,*,#7070,.F.);
#10111=ORIENTED_EDGE('',*,*,#7071,.F.);
#10112=ORIENTED_EDGE('',*,*,#7072,.T.);
#10113=ORIENTED_EDGE('',*,*,#7073,.T.);
#10114=ORIENTED_EDGE('',*,*,#7074,.F.);
#10115=ORIENTED_EDGE('',*,*,#7075,.F.);
#10116=ORIENTED_EDGE('',*,*,#7076,.T.);
#10117=ORIENTED_EDGE('',*,*,#7077,.T.);
#10118=ORIENTED_EDGE('',*,*,#7072,.F.);
#10119=ORIENTED_EDGE('',*,*,#7078,.F.);
#10120=ORIENTED_EDGE('',*,*,#7079,.T.);
#10121=ORIENTED_EDGE('',*,*,#7080,.T.);
#10122=ORIENTED_EDGE('',*,*,#7076,.F.);
#10123=ORIENTED_EDGE('',*,*,#7081,.F.);
#10124=ORIENTED_EDGE('',*,*,#7082,.T.);
#10125=ORIENTED_EDGE('',*,*,#7083,.T.);
#10126=ORIENTED_EDGE('',*,*,#7079,.F.);
#10127=ORIENTED_EDGE('',*,*,#7084,.F.);
#10128=ORIENTED_EDGE('',*,*,#7085,.T.);
#10129=ORIENTED_EDGE('',*,*,#7086,.T.);
#10130=ORIENTED_EDGE('',*,*,#7082,.F.);
#10131=ORIENTED_EDGE('',*,*,#7087,.F.);
#10132=ORIENTED_EDGE('',*,*,#7074,.T.);
#10133=ORIENTED_EDGE('',*,*,#7088,.T.);
#10134=ORIENTED_EDGE('',*,*,#7085,.F.);
#10135=ORIENTED_EDGE('',*,*,#7088,.F.);
#10136=ORIENTED_EDGE('',*,*,#7073,.F.);
#10137=ORIENTED_EDGE('',*,*,#7077,.F.);
#10138=ORIENTED_EDGE('',*,*,#7080,.F.);
#10139=ORIENTED_EDGE('',*,*,#7083,.F.);
#10140=ORIENTED_EDGE('',*,*,#7086,.F.);
#10141=ORIENTED_EDGE('',*,*,#7089,.F.);
#10142=ORIENTED_EDGE('',*,*,#7071,.T.);
#10143=ORIENTED_EDGE('',*,*,#7087,.T.);
#10144=ORIENTED_EDGE('',*,*,#7084,.T.);
#10145=ORIENTED_EDGE('',*,*,#7081,.T.);
#10146=ORIENTED_EDGE('',*,*,#7078,.T.);
#10147=ORIENTED_EDGE('',*,*,#7075,.T.);
#10148=ORIENTED_EDGE('',*,*,#7065,.F.);
#10149=ORIENTED_EDGE('',*,*,#7022,.F.);
#10150=ORIENTED_EDGE('',*,*,#7066,.F.);
#10151=ORIENTED_EDGE('',*,*,#7090,.T.);
#10152=ORIENTED_EDGE('',*,*,#7089,.T.);
#10153=ORIENTED_EDGE('',*,*,#7090,.F.);
#10154=ORIENTED_EDGE('',*,*,#7036,.T.);
#10155=ORIENTED_EDGE('',*,*,#7062,.T.);
#10156=ORIENTED_EDGE('',*,*,#7091,.F.);
#10157=ORIENTED_EDGE('',*,*,#7070,.T.);
#10158=ORIENTED_EDGE('',*,*,#7092,.F.);
#10159=ORIENTED_EDGE('',*,*,#7093,.T.);
#10160=ORIENTED_EDGE('',*,*,#7059,.T.);
#10161=ORIENTED_EDGE('',*,*,#7091,.T.);
#10162=ORIENTED_EDGE('',*,*,#7060,.T.);
#10163=ORIENTED_EDGE('',*,*,#7093,.F.);
#10164=ORIENTED_EDGE('',*,*,#7092,.T.);
#11597=PLANE('',#13152);
#11598=PLANE('',#13155);
#11599=PLANE('',#13160);
#11600=PLANE('',#13161);
#11601=PLANE('',#13162);
#11602=PLANE('',#13163);
#11603=PLANE('',#13164);
#11604=PLANE('',#13165);
#11605=PLANE('',#13166);
#11606=PLANE('',#13167);
#11607=PLANE('',#13174);
#12189=ADVANCED_FACE('',(#2222),#293,.T.);
#12190=ADVANCED_FACE('',(#2223),#294,.T.);
#12191=ADVANCED_FACE('',(#2224),#295,.T.);
#12192=ADVANCED_FACE('',(#2225),#296,.T.);
#12193=ADVANCED_FACE('',(#2226),#297,.T.);
#12194=ADVANCED_FACE('',(#2227),#298,.T.);
#12195=ADVANCED_FACE('',(#2228),#299,.T.);
#12196=ADVANCED_FACE('',(#2229),#300,.T.);
#12197=ADVANCED_FACE('',(#2230),#301,.T.);
#12198=ADVANCED_FACE('',(#2231),#302,.T.);
#12199=ADVANCED_FACE('',(#2232),#303,.T.);
#12200=ADVANCED_FACE('',(#2233),#304,.T.);
#12201=ADVANCED_FACE('',(#2234),#11597,.T.);
#12202=ADVANCED_FACE('',(#2235),#1330,.F.);
#12203=ADVANCED_FACE('',(#2236),#11598,.F.);
#12204=ADVANCED_FACE('',(#2237),#305,.T.);
#12205=ADVANCED_FACE('',(#2238),#1331,.F.);
#12206=ADVANCED_FACE('',(#2239),#11599,.F.);
#12207=ADVANCED_FACE('',(#2240),#11600,.F.);
#12208=ADVANCED_FACE('',(#2241),#11601,.F.);
#12209=ADVANCED_FACE('',(#2242),#11602,.F.);
#12210=ADVANCED_FACE('',(#2243),#11603,.F.);
#12211=ADVANCED_FACE('',(#2244),#11604,.F.);
#12212=ADVANCED_FACE('',(#2245),#11605,.F.);
#12213=ADVANCED_FACE('',(#2246,#1396),#11606,.T.);
#12214=ADVANCED_FACE('',(#2247),#435,.T.);
#12215=ADVANCED_FACE('',(#2248),#306,.T.);
#12216=ADVANCED_FACE('',(#2249),#436,.T.);
#12217=ADVANCED_FACE('',(#2250),#11607,.T.);
#12487=CLOSED_SHELL('',(#12189,#12190,#12191,#12192,#12193,#12194,#12195,
#12196,#12197,#12198,#12199,#12200,#12201,#12202,#12203,#12204,#12205,#12206,
#12207,#12208,#12209,#12210,#12211,#12212,#12213,#12214,#12215,#12216,#12217));
#13136=AXIS2_PLACEMENT_3D('',#25843,#14984,#14985);
#13137=AXIS2_PLACEMENT_3D('',#25844,#14986,#14987);
#13138=AXIS2_PLACEMENT_3D('',#25860,#14989,#14990);
#13139=AXIS2_PLACEMENT_3D('',#25868,#14991,#14992);
#13140=AXIS2_PLACEMENT_3D('',#25916,#14994,#14995);
#13141=AXIS2_PLACEMENT_3D('',#25964,#14997,#14998);
#13142=AXIS2_PLACEMENT_3D('',#26018,#15000,#15001);
#13143=AXIS2_PLACEMENT_3D('',#26066,#15003,#15004);
#13144=AXIS2_PLACEMENT_3D('',#26120,#15006,#15007);
#13145=AXIS2_PLACEMENT_3D('',#26129,#15009,#15010);
#13146=AXIS2_PLACEMENT_3D('',#26130,#15011,#15012);
#13147=AXIS2_PLACEMENT_3D('',#26146,#15014,#15015);
#13148=AXIS2_PLACEMENT_3D('',#26156,#15016,#15017);
#13149=AXIS2_PLACEMENT_3D('',#26181,#15019,#15020);
#13150=AXIS2_PLACEMENT_3D('',#26206,#15022,#15023);
#13151=AXIS2_PLACEMENT_3D('',#26231,#15025,#15026);
#13152=AXIS2_PLACEMENT_3D('',#26255,#15028,#15029);
#13153=AXIS2_PLACEMENT_3D('',#26310,#15030,#15031);
#13154=AXIS2_PLACEMENT_3D('',#26312,#15032,#15033);
#13155=AXIS2_PLACEMENT_3D('',#26611,#15034,#15035);
#13156=AXIS2_PLACEMENT_3D('',#26613,#15036,#15037);
#13157=AXIS2_PLACEMENT_3D('',#26614,#15038,#15039);
#13158=AXIS2_PLACEMENT_3D('',#26671,#15040,#15041);
#13159=AXIS2_PLACEMENT_3D('',#26672,#15042,#15043);
#13160=AXIS2_PLACEMENT_3D('',#26859,#15044,#15045);
#13161=AXIS2_PLACEMENT_3D('',#26868,#15050,#15051);
#13162=AXIS2_PLACEMENT_3D('',#26874,#15055,#15056);
#13163=AXIS2_PLACEMENT_3D('',#26880,#15060,#15061);
#13164=AXIS2_PLACEMENT_3D('',#26886,#15065,#15066);
#13165=AXIS2_PLACEMENT_3D('',#26892,#15070,#15071);
#13166=AXIS2_PLACEMENT_3D('',#26895,#15074,#15075);
#13167=AXIS2_PLACEMENT_3D('',#26896,#15076,#15077);
#13168=AXIS2_PLACEMENT_3D('',#26898,#15078,#15079);
#13169=AXIS2_PLACEMENT_3D('',#26899,#15080,#15081);
#13170=AXIS2_PLACEMENT_3D('',#26901,#15083,#15084);
#13171=AXIS2_PLACEMENT_3D('',#26902,#15085,#15086);
#13172=AXIS2_PLACEMENT_3D('',#26903,#15087,#15088);
#13173=AXIS2_PLACEMENT_3D('',#26905,#15089,#15090);
#13174=AXIS2_PLACEMENT_3D('',#26907,#15092,#15093);
#14984=DIRECTION('axis',(0.,0.,1.));
#14985=DIRECTION('refdir',(1.,0.,0.));
#14986=DIRECTION('center_axis',(-1.,0.,0.));
#14987=DIRECTION('ref_axis',(0.,0.,1.));
#14988=DIRECTION('',(1.,0.,0.));
#14989=DIRECTION('center_axis',(-1.,0.,0.));
#14990=DIRECTION('ref_axis',(0.,0.,1.));
#14991=DIRECTION('center_axis',(-1.,0.,0.));
#14992=DIRECTION('ref_axis',(0.,0.,1.));
#14993=DIRECTION('',(1.,0.,0.));
#14994=DIRECTION('center_axis',(-1.,0.,0.));
#14995=DIRECTION('ref_axis',(0.,0.,1.));
#14996=DIRECTION('',(1.,0.,0.));
#14997=DIRECTION('center_axis',(-1.,0.,0.));
#14998=DIRECTION('ref_axis',(0.,0.,1.));
#14999=DIRECTION('',(1.,0.,0.));
#15000=DIRECTION('center_axis',(-1.,0.,0.));
#15001=DIRECTION('ref_axis',(0.,0.,1.));
#15002=DIRECTION('',(1.,0.,0.));
#15003=DIRECTION('center_axis',(-1.,0.,0.));
#15004=DIRECTION('ref_axis',(0.,0.,1.));
#15005=DIRECTION('',(1.,0.,0.));
#15006=DIRECTION('center_axis',(-1.,0.,0.));
#15007=DIRECTION('ref_axis',(0.,-0.376634011382756,-0.92636214380216));
#15008=DIRECTION('',(-1.,0.,0.));
#15009=DIRECTION('center_axis',(-1.,0.,0.));
#15010=DIRECTION('ref_axis',(0.,1.36963031528353E-14,1.));
#15011=DIRECTION('center_axis',(-1.,0.,0.));
#15012=DIRECTION('ref_axis',(0.,1.36963031528353E-14,1.));
#15013=DIRECTION('',(-1.,0.,0.));
#15014=DIRECTION('center_axis',(-1.,0.,0.));
#15015=DIRECTION('ref_axis',(0.,1.36963031528353E-14,1.));
#15016=DIRECTION('center_axis',(-1.,0.,0.));
#15017=DIRECTION('ref_axis',(0.,1.36963031528353E-14,1.));
#15018=DIRECTION('',(-1.,0.,0.));
#15019=DIRECTION('center_axis',(-1.,0.,0.));
#15020=DIRECTION('ref_axis',(0.,1.36963031528353E-14,1.));
#15021=DIRECTION('',(-1.,0.,0.));
#15022=DIRECTION('center_axis',(-1.,0.,0.));
#15023=DIRECTION('ref_axis',(0.,1.36963031528353E-14,1.));
#15024=DIRECTION('',(-1.,0.,0.));
#15025=DIRECTION('center_axis',(-1.,0.,0.));
#15026=DIRECTION('ref_axis',(0.,1.36963031528353E-14,1.));
#15027=DIRECTION('',(-1.,0.,0.));
#15028=DIRECTION('center_axis',(1.,0.,0.));
#15029=DIRECTION('ref_axis',(0.,0.,-1.));
#15030=DIRECTION('center_axis',(1.,0.,0.));
#15031=DIRECTION('ref_axis',(0.,0.,1.));
#15032=DIRECTION('center_axis',(1.,0.,0.));
#15033=DIRECTION('ref_axis',(0.,0.,1.));
#15034=DIRECTION('center_axis',(1.,0.,0.));
#15035=DIRECTION('ref_axis',(0.,0.,-1.));
#15036=DIRECTION('center_axis',(-1.,0.,0.));
#15037=DIRECTION('ref_axis',(0.,0.,1.));
#15038=DIRECTION('center_axis',(-1.,0.,0.));
#15039=DIRECTION('ref_axis',(0.,0.,1.));
#15040=DIRECTION('center_axis',(1.,0.,0.));
#15041=DIRECTION('ref_axis',(0.,1.36963031528353E-14,1.));
#15042=DIRECTION('center_axis',(-1.,0.,0.));
#15043=DIRECTION('ref_axis',(0.,0.457593006249823,0.88916176291564));
#15044=DIRECTION('center_axis',(0.,0.866025403784439,0.5));
#15045=DIRECTION('ref_axis',(0.,0.5,-0.866025403784439));
#15046=DIRECTION('',(0.,0.5,-0.866025403784439));
#15047=DIRECTION('',(-1.,0.,0.));
#15048=DIRECTION('',(0.,0.5,-0.866025403784439));
#15049=DIRECTION('',(-1.,0.,0.));
#15050=DIRECTION('center_axis',(0.,0.,1.));
#15051=DIRECTION('ref_axis',(0.,1.,0.));
#15052=DIRECTION('',(0.,1.,0.));
#15053=DIRECTION('',(-1.,0.,0.));
#15054=DIRECTION('',(0.,1.,0.));
#15055=DIRECTION('center_axis',(0.,-0.866025403784439,0.5));
#15056=DIRECTION('ref_axis',(0.,0.5,0.866025403784439));
#15057=DIRECTION('',(0.,0.5,0.866025403784439));
#15058=DIRECTION('',(-1.,0.,0.));
#15059=DIRECTION('',(0.,0.5,0.866025403784439));
#15060=DIRECTION('center_axis',(0.,-0.866025403784439,-0.499999999999999));
#15061=DIRECTION('ref_axis',(0.,-0.499999999999999,0.866025403784439));
#15062=DIRECTION('',(0.,-0.499999999999999,0.866025403784439));
#15063=DIRECTION('',(-1.,0.,0.));
#15064=DIRECTION('',(0.,-0.499999999999999,0.866025403784439));
#15065=DIRECTION('center_axis',(0.,0.,-1.));
#15066=DIRECTION('ref_axis',(0.,-1.,0.));
#15067=DIRECTION('',(0.,-1.,0.));
#15068=DIRECTION('',(-1.,0.,0.));
#15069=DIRECTION('',(0.,-1.,0.));
#15070=DIRECTION('center_axis',(0.,0.866025403784439,-0.5));
#15071=DIRECTION('ref_axis',(0.,-0.5,-0.866025403784439));
#15072=DIRECTION('',(0.,-0.5,-0.866025403784439));
#15073=DIRECTION('',(0.,-0.5,-0.866025403784439));
#15074=DIRECTION('center_axis',(-1.,0.,0.));
#15075=DIRECTION('ref_axis',(0.,0.,1.));
#15076=DIRECTION('center_axis',(1.,0.,0.));
#15077=DIRECTION('ref_axis',(0.,0.,-1.));
#15078=DIRECTION('center_axis',(-1.,0.,0.));
#15079=DIRECTION('ref_axis',(0.,0.,1.));
#15080=DIRECTION('center_axis',(-1.,0.,0.));
#15081=DIRECTION('ref_axis',(0.,0.,1.));
#15082=DIRECTION('',(0.70710678118655,8.6595605623549E-17,0.707106781186545));
#15083=DIRECTION('center_axis',(-1.,0.,0.));
#15084=DIRECTION('ref_axis',(0.,-0.953985326168334,0.299853293221031));
#15085=DIRECTION('center_axis',(1.,0.,0.));
#15086=DIRECTION('ref_axis',(0.,0.,1.));
#15087=DIRECTION('center_axis',(1.,0.,0.));
#15088=DIRECTION('ref_axis',(0.,0.,1.));
#15089=DIRECTION('center_axis',(-1.,0.,0.));
#15090=DIRECTION('ref_axis',(0.,0.,1.));
#15091=DIRECTION('',(0.707106781186549,-8.65956056235492E-17,-0.707106781186546));
#15092=DIRECTION('center_axis',(-1.,0.,0.));
#15093=DIRECTION('ref_axis',(0.,0.,1.));
#25843=CARTESIAN_POINT('',(0.,0.,0.));
#25844=CARTESIAN_POINT('Origin',(0.7225,0.,2.35));
#25845=CARTESIAN_POINT('',(0.902013030787577,0.000156006175312973,2.15447233455283));
#25846=CARTESIAN_POINT('',(0.912186969212423,0.000188656559950066,2.15445617438948));
#25847=CARTESIAN_POINT('',(0.7225,-2.39295984553393E-17,2.1546));
#25848=CARTESIAN_POINT('',(0.9246,0.175480723124223,2.43625468886433));
#25849=CARTESIAN_POINT('Ctrl Pts',(0.902013030787577,0.000156006175312973,
2.15447233455283));
#25850=CARTESIAN_POINT('Ctrl Pts',(0.902605775122933,0.0105315582112279,
2.15438573053182));
#25851=CARTESIAN_POINT('Ctrl Pts',(0.90319851945829,0.0208939809769666,
2.15514242031383));
#25852=CARTESIAN_POINT('Ctrl Pts',(0.903791263793647,0.0311127383116308,
2.1567873079189));
#25853=CARTESIAN_POINT('Ctrl Pts',(0.90744260916311,0.0940609776282298,
2.16691992729932));
#25854=CARTESIAN_POINT('Ctrl Pts',(0.911093954532574,0.151557625733869,
2.21075648930218));
#25855=CARTESIAN_POINT('Ctrl Pts',(0.914745299902037,0.178037552885034,
2.26877728473645));
#25856=CARTESIAN_POINT('Ctrl Pts',(0.918030199934691,0.201859981267461,
2.32097517168809));
#25857=CARTESIAN_POINT('Ctrl Pts',(0.921315099967346,0.20057890417809,2.38465312392714));
#25858=CARTESIAN_POINT('Ctrl Pts',(0.9246,0.175579315085691,2.4363567917616));
#25859=CARTESIAN_POINT('',(0.9246,0.175382131162755,2.26384741403295));
#25860=CARTESIAN_POINT('Origin',(0.9246,0.,2.35));
#25861=CARTESIAN_POINT('Ctrl Pts',(0.9246,0.175382131162755,2.26384741403295));
#25862=CARTESIAN_POINT('Ctrl Pts',(0.920948654630537,0.147146138548361,
2.20636697389733));
#25863=CARTESIAN_POINT('Ctrl Pts',(0.917297309261073,0.0887096319793009,
2.16430051430661));
#25864=CARTESIAN_POINT('Ctrl Pts',(0.91364596389161,0.0255879622251572,
2.15600165398185));
#25865=CARTESIAN_POINT('Ctrl Pts',(0.913159632331881,0.0171806336933338,
2.15489630861533));
#25866=CARTESIAN_POINT('Ctrl Pts',(0.912673300772152,0.0086901893208547,
2.15439000799688));
#25867=CARTESIAN_POINT('Ctrl Pts',(0.912186969212423,0.000188656559950066,
2.15445617438948));
#25868=CARTESIAN_POINT('Origin',(0.7225,0.,2.35));
#25869=CARTESIAN_POINT('',(0.832013030787577,-5.13316928911073E-5,2.15488450746355));
#25870=CARTESIAN_POINT('',(0.842186969212423,-2.25216307721818E-5,2.15489585068442));
#25871=CARTESIAN_POINT('',(0.7225,-2.39295984553393E-17,2.1546));
#25872=CARTESIAN_POINT('Ctrl Pts',(0.832013030787577,-5.13316928911073E-5,
2.15488450746355));
#25873=CARTESIAN_POINT('Ctrl Pts',(0.834031036239487,0.0354651555565149,
2.15497065566532));
#25874=CARTESIAN_POINT('Ctrl Pts',(0.836049041691397,0.0710236125991935,
2.16426571469804));
#25875=CARTESIAN_POINT('Ctrl Pts',(0.838067047143308,0.101189284396635,
2.18248793521357));
#25876=CARTESIAN_POINT('Ctrl Pts',(0.841718392512771,0.155770547261944,
2.21545891675267));
#25877=CARTESIAN_POINT('Ctrl Pts',(0.845369737882234,0.192696543426469,
2.27765624603097));
#25878=CARTESIAN_POINT('Ctrl Pts',(0.849021083251698,0.195511659694429,
2.34136106334354));
#25879=CARTESIAN_POINT('Ctrl Pts',(0.852672428621161,0.198326775962389,
2.40506588065611));
#25880=CARTESIAN_POINT('Ctrl Pts',(0.856323773990624,0.167031012333786,
2.47027818600294));
#25881=CARTESIAN_POINT('Ctrl Pts',(0.859975119360087,0.115569820078586,
2.50793461140361));
#25882=CARTESIAN_POINT('Ctrl Pts',(0.86362646472955,0.0641086278233862,
2.54559103680428));
#25883=CARTESIAN_POINT('Ctrl Pts',(0.867277810099014,-0.00751799305840972,
2.55569158225879));
#25884=CARTESIAN_POINT('Ctrl Pts',(0.870929155468477,-0.0673847305716984,
2.53373589439266));
#25885=CARTESIAN_POINT('Ctrl Pts',(0.874580500837941,-0.127251468084987,
2.51178020652652));
#25886=CARTESIAN_POINT('Ctrl Pts',(0.878231846207404,-0.175358322229768,
2.45776828533975));
#25887=CARTESIAN_POINT('Ctrl Pts',(0.881883191576868,-0.190273413583082,
2.39576915322462));
#25888=CARTESIAN_POINT('Ctrl Pts',(0.885534536946331,-0.205188504936396,
2.33377002110949));
#25889=CARTESIAN_POINT('Ctrl Pts',(0.889185882315794,-0.186911833498241,
2.26378367806601));
#25890=CARTESIAN_POINT('Ctrl Pts',(0.892837227685257,-0.143573582515385,
2.21700484492326));
#25891=CARTESIAN_POINT('Ctrl Pts',(0.895895828719363,-0.107270684306657,
2.17781989446053));
#25892=CARTESIAN_POINT('Ctrl Pts',(0.89895442975347,-0.0533825471157545,
2.15491921718409));
#25893=CARTESIAN_POINT('Ctrl Pts',(0.902013030787577,0.000156006175312973,
2.15447233455283));
#25894=CARTESIAN_POINT('Ctrl Pts',(0.912186969212423,0.000188656559950066,
2.15445617438948));
#25895=CARTESIAN_POINT('Ctrl Pts',(0.909021955402688,-0.0551387595903964,
2.15488678092139));
#25896=CARTESIAN_POINT('Ctrl Pts',(0.905856941592954,-0.110935804562971,
2.17956320188895));
#25897=CARTESIAN_POINT('Ctrl Pts',(0.90269192778322,-0.147349415349169,
2.22115976531861));
#25898=CARTESIAN_POINT('Ctrl Pts',(0.899040582413757,-0.189358290230125,
2.2691479980389));
#25899=CARTESIAN_POINT('Ctrl Pts',(0.895389237044293,-0.205569207052808,
2.33965572453828));
#25900=CARTESIAN_POINT('Ctrl Pts',(0.89173789167483,-0.188870701167725,
2.40120859986922));
#25901=CARTESIAN_POINT('Ctrl Pts',(0.888086546305367,-0.172172195282643,
2.46276147520016));
#25902=CARTESIAN_POINT('Ctrl Pts',(0.884435200935903,-0.122564266689796,
2.51535949936266));
#25903=CARTESIAN_POINT('Ctrl Pts',(0.88078385556644,-0.0620996521231525,
2.53558762972075));
#25904=CARTESIAN_POINT('Ctrl Pts',(0.877132510196977,-0.00163503755650911,
2.55581576007883));
#25905=CARTESIAN_POINT('Ctrl Pts',(0.873481164827514,0.06968626298393,2.54367399663249));
#25906=CARTESIAN_POINT('Ctrl Pts',(0.86982981945805,0.120050756860153,2.50456030751575));
#25907=CARTESIAN_POINT('Ctrl Pts',(0.866178474088587,0.170415250736377,
2.465446618399));
#25908=CARTESIAN_POINT('Ctrl Pts',(0.862527128719124,0.199822937948385,
2.39936100361186));
#25909=CARTESIAN_POINT('Ctrl Pts',(0.85887578334966,0.195182096220547,2.33576215814722));
#25910=CARTESIAN_POINT('Ctrl Pts',(0.855224437980197,0.190541254492709,
2.27216331268259));
#25911=CARTESIAN_POINT('Ctrl Pts',(0.851573092610733,0.151851883825026,
2.21105123654046));
#25912=CARTESIAN_POINT('Ctrl Pts',(0.84792174724127,0.096349247276285,2.17965802669765));
#25913=CARTESIAN_POINT('Ctrl Pts',(0.846010154564988,0.0672918936695139,
2.16322270657636));
#25914=CARTESIAN_POINT('Ctrl Pts',(0.844098561888705,0.0336262801083577,
2.15493287481085));
#25915=CARTESIAN_POINT('Ctrl Pts',(0.842186969212423,-2.25216307721818E-5,
2.15489585068442));
#25916=CARTESIAN_POINT('Origin',(0.7225,0.,2.35));
#25917=CARTESIAN_POINT('',(0.762013030787577,-6.2003443803138E-5,2.15432352696516));
#25918=CARTESIAN_POINT('',(0.772186969212424,-9.0396132758989E-5,2.15435402400981));
#25919=CARTESIAN_POINT('',(0.7225,-2.39295984553393E-17,2.1546));
#25920=CARTESIAN_POINT('Ctrl Pts',(0.762013030787577,-6.2003443803138E-5,
2.15432352696516));
#25921=CARTESIAN_POINT('Ctrl Pts',(0.765456297356041,0.0600926660966559,
2.15457840373805));
#25922=CARTESIAN_POINT('Ctrl Pts',(0.768899563924504,0.12046670050001,2.18446056958971));
#25923=CARTESIAN_POINT('Ctrl Pts',(0.772342830492968,0.156551060252226,
2.23256357411178));
#25924=CARTESIAN_POINT('Ctrl Pts',(0.775994175862431,0.194816020943342,
2.28357347396316));
#25925=CARTESIAN_POINT('Ctrl Pts',(0.779645521231895,0.205766923289551,
2.35507294634627));
#25926=CARTESIAN_POINT('Ctrl Pts',(0.783296866601358,0.184523355575946,
2.41519721875575));
#25927=CARTESIAN_POINT('Ctrl Pts',(0.786948211970822,0.163279787862341,
2.47532149116522));
#25928=CARTESIAN_POINT('Ctrl Pts',(0.790599557340285,0.109841750088923,
2.52407056360106));
#25929=CARTESIAN_POINT('Ctrl Pts',(0.794250902709748,0.0480246460538724,
2.53971869511427));
#25930=CARTESIAN_POINT('Ctrl Pts',(0.797902248079211,-0.0137924579811777,
2.55536682662749));
#25931=CARTESIAN_POINT('Ctrl Pts',(0.801553593448674,-0.0839886282778601,
2.53791401721809));
#25932=CARTESIAN_POINT('Ctrl Pts',(0.805204938818138,-0.131279857599735,
2.49513838326637));
#25933=CARTESIAN_POINT('Ctrl Pts',(0.808856284187601,-0.178571086921609,
2.45236274931465));
#25934=CARTESIAN_POINT('Ctrl Pts',(0.812507629557065,-0.202957375268676,
2.38426429082061));
#25935=CARTESIAN_POINT('Ctrl Pts',(0.816158974926528,-0.193570748439729,
2.32119203719827));
#25936=CARTESIAN_POINT('Ctrl Pts',(0.819810320295991,-0.184184121610782,
2.25811978357594));
#25937=CARTESIAN_POINT('Ctrl Pts',(0.823461665665454,-0.141024579605821,
2.20007373482531));
#25938=CARTESIAN_POINT('Ctrl Pts',(0.827113011034917,-0.0833265438202942,
2.17292302734994));
#25939=CARTESIAN_POINT('Ctrl Pts',(0.82874635095247,-0.0575167407266036,
2.1607778233711));
#25940=CARTESIAN_POINT('Ctrl Pts',(0.830379690870024,-0.0287977834434585,
2.15481478054748));
#25941=CARTESIAN_POINT('Ctrl Pts',(0.832013030787577,-5.13316928911073E-5,
2.15488450746355));
#25942=CARTESIAN_POINT('Ctrl Pts',(0.842186969212423,-2.25216307721818E-5,
2.15489585068442));
#25943=CARTESIAN_POINT('Ctrl Pts',(0.840447216519242,-0.0306465108175295,
2.15486215479069));
#25944=CARTESIAN_POINT('Ctrl Pts',(0.838707463826061,-0.0612565748792723,
2.16166420685548));
#25945=CARTESIAN_POINT('Ctrl Pts',(0.836967711132881,-0.0883661713810414,
2.17538290794441));
#25946=CARTESIAN_POINT('Ctrl Pts',(0.833316365763417,-0.145263051059827,
2.20417534257747));
#25947=CARTESIAN_POINT('Ctrl Pts',(0.829665020393954,-0.1867409079876,2.26343455538708));
#25948=CARTESIAN_POINT('Ctrl Pts',(0.82601367502449,-0.194316387043185,
2.32674994840334));
#25949=CARTESIAN_POINT('Ctrl Pts',(0.822362329655027,-0.20189186609877,
2.3900653414196));
#25950=CARTESIAN_POINT('Ctrl Pts',(0.818710984285564,-0.175564967282168,
2.4574369146425));
#25951=CARTESIAN_POINT('Ctrl Pts',(0.815059638916101,-0.127067715562319,
2.49883998978819));
#25952=CARTESIAN_POINT('Ctrl Pts',(0.811408293546638,-0.0785704638424689,
2.54024306493387));
#25953=CARTESIAN_POINT('Ctrl Pts',(0.807756948177174,-0.00790285921937169,
2.55567764200234));
#25954=CARTESIAN_POINT('Ctrl Pts',(0.804105602807711,0.053440578734723,
2.53826485429949));
#25955=CARTESIAN_POINT('Ctrl Pts',(0.800454257438247,0.114784016688818,
2.52085206659665));
#25956=CARTESIAN_POINT('Ctrl Pts',(0.796802912068784,0.16680328797391,2.4705919141225));
#25957=CARTESIAN_POINT('Ctrl Pts',(0.793151566699321,0.186315490867467,
2.40988367637621));
#25958=CARTESIAN_POINT('Ctrl Pts',(0.789500221329858,0.205827693761024,
2.34917543862993));
#25959=CARTESIAN_POINT('Ctrl Pts',(0.785848875960394,0.192832828263045,
2.27801911561151));
#25960=CARTESIAN_POINT('Ctrl Pts',(0.782197530590931,0.153122122420705,
2.22812649775847));
#25961=CARTESIAN_POINT('Ctrl Pts',(0.778860676798095,0.116831712722845,
2.18253114747751));
#25962=CARTESIAN_POINT('Ctrl Pts',(0.775523823005259,0.058229361212525,
2.15469434591714));
#25963=CARTESIAN_POINT('Ctrl Pts',(0.772186969212424,-9.0396132758989E-5,
2.15435402400981));
#25964=CARTESIAN_POINT('Origin',(0.7225,0.,2.35));
#25965=CARTESIAN_POINT('',(0.692013030787577,0.000139690484509278,2.15476836676823));
#25966=CARTESIAN_POINT('',(0.702186969212423,0.000153231897286442,2.15472339864344));
#25967=CARTESIAN_POINT('',(0.7225,-2.39295984553393E-17,2.1546));
#25968=CARTESIAN_POINT('Ctrl Pts',(0.692013030787577,0.000139690484509278,
2.15476836676823));
#25969=CARTESIAN_POINT('Ctrl Pts',(0.693230213103131,0.0215297149542501,
2.15462161982292));
#25970=CARTESIAN_POINT('Ctrl Pts',(0.694447395418685,0.0428763997647126,
2.15787240017079));
#25971=CARTESIAN_POINT('Ctrl Pts',(0.695664577734239,0.0630016027810242,
2.16471549811569));
#25972=CARTESIAN_POINT('Ctrl Pts',(0.699315923103702,0.123373878901117,
2.18524365866698));
#25973=CARTESIAN_POINT('Ctrl Pts',(0.702967268473165,0.172754032575755,
2.23809910815419));
#25974=CARTESIAN_POINT('Ctrl Pts',(0.706618613842629,0.189135076720051,
2.29972604120156));
#25975=CARTESIAN_POINT('Ctrl Pts',(0.710269959212092,0.205516120864348,
2.36135297424894));
#25976=CARTESIAN_POINT('Ctrl Pts',(0.713921304581555,0.188898055478303,
2.43175139085649));
#25977=CARTESIAN_POINT('Ctrl Pts',(0.717572649951018,0.146686965318226,
2.4795472189561));
#25978=CARTESIAN_POINT('Ctrl Pts',(0.721223995320482,0.104475875158149,
2.52734304705571));
#25979=CARTESIAN_POINT('Ctrl Pts',(0.724875340689945,0.0366717602240398,
2.55253628664739));
#25980=CARTESIAN_POINT('Ctrl Pts',(0.728526686059409,-0.0265074936359106,
2.54389920290807));
#25981=CARTESIAN_POINT('Ctrl Pts',(0.732178031428872,-0.0896867474958605,
2.53526211916876));
#25982=CARTESIAN_POINT('Ctrl Pts',(0.735829376798335,-0.148241140281651,
2.49279471209846));
#25983=CARTESIAN_POINT('Ctrl Pts',(0.739480722167799,-0.176075055463372,
2.43542319913709));
#25984=CARTESIAN_POINT('Ctrl Pts',(0.743132067537262,-0.203908970645092,
2.37805168617571));
#25985=CARTESIAN_POINT('Ctrl Pts',(0.746783412906725,-0.201022408222742,
2.30577606732327));
#25986=CARTESIAN_POINT('Ctrl Pts',(0.750434758276188,-0.168701809129991,
2.25080701975543));
#25987=CARTESIAN_POINT('Ctrl Pts',(0.754086103645651,-0.13638121003724,
2.1958379721876));
#25988=CARTESIAN_POINT('Ctrl Pts',(0.757737449015115,-0.0746265742740901,
2.15817549590436));
#25989=CARTESIAN_POINT('Ctrl Pts',(0.761388794384578,-0.0109597468745028,
2.15460442142256));
#25990=CARTESIAN_POINT('Ctrl Pts',(0.761596873185578,-0.00733157266245871,
2.15440091700945));
#25991=CARTESIAN_POINT('Ctrl Pts',(0.761804951986577,-0.00369718859825643,
2.15430812459876));
#25992=CARTESIAN_POINT('Ctrl Pts',(0.762013030787577,-6.2003443803138E-5,
2.15432352696516));
#25993=CARTESIAN_POINT('Ctrl Pts',(0.772186969212424,-9.0396132758989E-5,
2.15435402400981));
#25994=CARTESIAN_POINT('Ctrl Pts',(0.771872477635796,-0.00558691278428774,
2.15432194937309));
#25995=CARTESIAN_POINT('Ctrl Pts',(0.771557986059169,-0.0110809192442294,
2.15453411697643));
#25996=CARTESIAN_POINT('Ctrl Pts',(0.771243494482542,-0.0165534999638003,
2.15499867915844));
#25997=CARTESIAN_POINT('Ctrl Pts',(0.767592149113078,-0.0800918703192643,
2.16039239109913));
#25998=CARTESIAN_POINT('Ctrl Pts',(0.763940803743614,-0.140742064843491,
2.19980872766818));
#25999=CARTESIAN_POINT('Ctrl Pts',(0.760289458374151,-0.171474475734038,
2.25568121175218));
#26000=CARTESIAN_POINT('Ctrl Pts',(0.756638113004688,-0.202206886624584,
2.31155369583617));
#26001=CARTESIAN_POINT('Ctrl Pts',(0.752986767635225,-0.203021513881451,
2.38388232743512));
#26002=CARTESIAN_POINT('Ctrl Pts',(0.749335422265761,-0.173555291090547,
2.44043280991382));
#26003=CARTESIAN_POINT('Ctrl Pts',(0.745684076896298,-0.144089068299643,
2.49698329239251));
#26004=CARTESIAN_POINT('Ctrl Pts',(0.742032731526834,-0.0843419954609685,
2.53775562575096));
#26005=CARTESIAN_POINT('Ctrl Pts',(0.738381386157371,-0.0209412306637257,
2.54457902408615));
#26006=CARTESIAN_POINT('Ctrl Pts',(0.734730040787908,0.0424595341335172,
2.55140242242134));
#26007=CARTESIAN_POINT('Ctrl Pts',(0.731078695418445,0.109513990889328,
2.52427688573327));
#26008=CARTESIAN_POINT('Ctrl Pts',(0.727427350048982,0.150338352188362,
2.47529130523621));
#26009=CARTESIAN_POINT('Ctrl Pts',(0.723776004679519,0.191162713487395,
2.42630572473914));
#26010=CARTESIAN_POINT('Ctrl Pts',(0.720124659310055,0.205756979329652,
2.35546010043307));
#26011=CARTESIAN_POINT('Ctrl Pts',(0.716473313940591,0.187617001058584,
2.29432781126921));
#26012=CARTESIAN_POINT('Ctrl Pts',(0.712821968571128,0.169477022787516,
2.23319552210535));
#26013=CARTESIAN_POINT('Ctrl Pts',(0.709170623201665,0.118602800403123,
2.1817765680837));
#26014=CARTESIAN_POINT('Ctrl Pts',(0.705519277832202,0.0576671708412165,
2.16298655371481));
#26015=CARTESIAN_POINT('Ctrl Pts',(0.704408508292276,0.0391300470238821,
2.15727047552887));
#26016=CARTESIAN_POINT('Ctrl Pts',(0.70329773875235,0.0196618135696035,
2.15457396703312));
#26017=CARTESIAN_POINT('Ctrl Pts',(0.702186969212423,0.000153231897286442,
2.15472339864344));
#26018=CARTESIAN_POINT('Origin',(0.7225,0.,2.35));
#26019=CARTESIAN_POINT('',(0.622013030787577,-0.000161508074393329,2.15467656254574));
#26020=CARTESIAN_POINT('',(0.632186969212423,-0.000152729840347416,2.15472545757722));
#26021=CARTESIAN_POINT('',(0.7225,-2.39295984553393E-17,2.1546));
#26022=CARTESIAN_POINT('Ctrl Pts',(0.622013030787577,-0.000161508074393329,
2.15467656254574));
#26023=CARTESIAN_POINT('Ctrl Pts',(0.624655474219684,0.0462195525262236,
2.15505898169449));
#26024=CARTESIAN_POINT('Ctrl Pts',(0.627297917651792,0.0928466454266734,
2.17165020966846));
#26025=CARTESIAN_POINT('Ctrl Pts',(0.629940361083899,0.127796252092552,
2.2017850173673));
#26026=CARTESIAN_POINT('Ctrl Pts',(0.633591706453363,0.17608984389226,2.2434254889149));
#26027=CARTESIAN_POINT('Ctrl Pts',(0.637243051822826,0.202086571273201,
2.31092592336927));
#26028=CARTESIAN_POINT('Ctrl Pts',(0.640894397192289,0.194200323183497,
2.37420333909549));
#26029=CARTESIAN_POINT('Ctrl Pts',(0.644545742561752,0.186314075093794,
2.43748075482171));
#26030=CARTESIAN_POINT('Ctrl Pts',(0.648197087931216,0.144544851533446,
2.49653515181977));
#26031=CARTESIAN_POINT('Ctrl Pts',(0.651848433300679,0.0875078611215212,
2.52504830080363));
#26032=CARTESIAN_POINT('Ctrl Pts',(0.655499778670142,0.0304708707095967,
2.5535614497875));
#26033=CARTESIAN_POINT('Ctrl Pts',(0.659151124039606,-0.0418338865539044,
2.55153335075717));
#26034=CARTESIAN_POINT('Ctrl Pts',(0.662802469409069,-0.0971828214413289,
2.51986774421674));
#26035=CARTESIAN_POINT('Ctrl Pts',(0.666453814778532,-0.152531756328753,
2.48820213767631));
#26036=CARTESIAN_POINT('Ctrl Pts',(0.670105160147996,-0.190924868840101,
2.42689902362578));
#26037=CARTESIAN_POINT('Ctrl Pts',(0.673756505517459,-0.195251673282228,
2.36327908072691));
#26038=CARTESIAN_POINT('Ctrl Pts',(0.677407850886922,-0.199578477724354,
2.29965913782805));
#26039=CARTESIAN_POINT('Ctrl Pts',(0.681059196256386,-0.16983897409726,
2.23372236608085));
#26040=CARTESIAN_POINT('Ctrl Pts',(0.684710541625849,-0.119287023000938,
2.19485441601494));
#26041=CARTESIAN_POINT('Ctrl Pts',(0.687144704679758,-0.0855866525317966,
2.16894316455599));
#26042=CARTESIAN_POINT('Ctrl Pts',(0.689578867733667,-0.0426368160594284,
2.15506183635612));
#26043=CARTESIAN_POINT('Ctrl Pts',(0.692013030787577,0.000139690484509278,
2.15476836676823));
#26044=CARTESIAN_POINT('Ctrl Pts',(0.702186969212423,0.000153231897286442,
2.15472339864344));
#26045=CARTESIAN_POINT('Ctrl Pts',(0.699646393382886,-0.0444672130138438,
2.15506518181601));
#26046=CARTESIAN_POINT('Ctrl Pts',(0.697105817553348,-0.0892987348503382,
2.17029516368888));
#26047=CARTESIAN_POINT('Ctrl Pts',(0.694565241723811,-0.123683081253107,
2.19833580937399));
#26048=CARTESIAN_POINT('Ctrl Pts',(0.690913896354348,-0.173100667046107,
2.23863615411818));
#26049=CARTESIAN_POINT('Ctrl Pts',(0.687262550984885,-0.200938801892689,
2.30539791832267));
#26050=CARTESIAN_POINT('Ctrl Pts',(0.683611205615422,-0.194791014914288,
2.36886775727776));
#26051=CARTESIAN_POINT('Ctrl Pts',(0.679959860245959,-0.188643227935887,
2.43233759623284));
#26052=CARTESIAN_POINT('Ctrl Pts',(0.676308514876495,-0.148509519132504,
2.49251550993851));
#26053=CARTESIAN_POINT('Ctrl Pts',(0.672657169507032,-0.0922760620207351,
2.52258232978025));
#26054=CARTESIAN_POINT('Ctrl Pts',(0.669005824137568,-0.0360426049089654,
2.55264914962198));
#26055=CARTESIAN_POINT('Ctrl Pts',(0.665354478768105,0.0362906005111901,
2.55260487559978));
#26056=CARTESIAN_POINT('Ctrl Pts',(0.661703133398642,0.0924872190443799,
2.52246925511011));
#26057=CARTESIAN_POINT('Ctrl Pts',(0.658051788029179,0.148683837577569,
2.49233363462045));
#26058=CARTESIAN_POINT('Ctrl Pts',(0.654400442659716,0.188743869223793,
2.43210666766332));
#26059=CARTESIAN_POINT('Ctrl Pts',(0.650749097290252,0.19481396515396,2.36862934437913));
#26060=CARTESIAN_POINT('Ctrl Pts',(0.647097751920789,0.200884061084127,
2.30515202109494));
#26061=CARTESIAN_POINT('Ctrl Pts',(0.643446406551326,0.172964221298237,
2.23842434148368));
#26062=CARTESIAN_POINT('Ctrl Pts',(0.639795061181862,0.123497355969801,
2.19818452650765));
#26063=CARTESIAN_POINT('Ctrl Pts',(0.637259030525382,0.089140297335463,
2.17023608721628));
#26064=CARTESIAN_POINT('Ctrl Pts',(0.634722999868903,0.0443890523714131,
2.15506527237943));
#26065=CARTESIAN_POINT('Ctrl Pts',(0.632186969212423,-0.000152729840347416,
2.15472545757722));
#26066=CARTESIAN_POINT('Origin',(0.7225,0.,2.35));
#26067=CARTESIAN_POINT('',(0.552013030787577,0.000119548669269599,2.15439909884273));
#26068=CARTESIAN_POINT('',(0.562186969212423,8.98932785041182E-5,2.15435395233057));
#26069=CARTESIAN_POINT('',(0.7225,-2.39295984553393E-17,2.1546));
#26070=CARTESIAN_POINT('Ctrl Pts',(0.552013030787577,0.000119548669269599,
2.15439909884273));
#26071=CARTESIAN_POINT('Ctrl Pts',(0.552429389966775,0.00740179500524078,
2.1543504652939));
#26072=CARTESIAN_POINT('Ctrl Pts',(0.552845749145972,0.0146785211588285,
2.1547249528878));
#26073=CARTESIAN_POINT('Ctrl Pts',(0.55326210832517,0.0219052057459278,
2.15554007694822));
#26074=CARTESIAN_POINT('Ctrl Pts',(0.556913453694633,0.0852810663538896,
2.16268847096059));
#26075=CARTESIAN_POINT('Ctrl Pts',(0.560564799064096,0.144808347695821,
2.2037251799862));
#26076=CARTESIAN_POINT('Ctrl Pts',(0.564216144433559,0.173992070839574,
2.26041257816284));
#26077=CARTESIAN_POINT('Ctrl Pts',(0.567867489803023,0.203175793983327,
2.31709997633948));
#26078=CARTESIAN_POINT('Ctrl Pts',(0.571518835172486,0.202015958928901,
2.38943806366715));
#26079=CARTESIAN_POINT('Ctrl Pts',(0.575170180541949,0.171012158196446,
2.44516263247295));
#26080=CARTESIAN_POINT('Ctrl Pts',(0.578821525911413,0.140008357463991,
2.50088720127875));
#26081=CARTESIAN_POINT('Ctrl Pts',(0.582472871280876,0.0791605910535053,
2.53999825156269));
#26082=CARTESIAN_POINT('Ctrl Pts',(0.58612421665034,0.0155953124083451,
2.54507837792627));
#26083=CARTESIAN_POINT('Ctrl Pts',(0.589775562019803,-0.0479699662368153,
2.55015850428984));
#26084=CARTESIAN_POINT('Ctrl Pts',(0.593426907389266,-0.11425275711665,
2.52120770673306));
#26085=CARTESIAN_POINT('Ctrl Pts',(0.597078252758729,-0.153717611658953,
2.47112174316925));
#26086=CARTESIAN_POINT('Ctrl Pts',(0.600729598128193,-0.193182466201255,
2.42103577960544));
#26087=CARTESIAN_POINT('Ctrl Pts',(0.604380943497656,-0.205829384406025,
2.34981465003461));
#26088=CARTESIAN_POINT('Ctrl Pts',(0.608032288867119,-0.186019835097296,
2.28920241992824));
#26089=CARTESIAN_POINT('Ctrl Pts',(0.611683634236583,-0.166210285788567,
2.22859018982187));
#26090=CARTESIAN_POINT('Ctrl Pts',(0.615334979606046,-0.113944268966339,
2.17858685917995));
#26091=CARTESIAN_POINT('Ctrl Pts',(0.618986324975509,-0.0525160324459869,
2.1614754481794));
#26092=CARTESIAN_POINT('Ctrl Pts',(0.619995226912865,-0.0355428183118095,
2.15674740030595));
#26093=CARTESIAN_POINT('Ctrl Pts',(0.621004128850221,-0.0178700960153893,
2.15453055244942));
#26094=CARTESIAN_POINT('Ctrl Pts',(0.622013030787577,-0.000161508074393329,
2.15467656254574));
#26095=CARTESIAN_POINT('Ctrl Pts',(0.632186969212423,-0.000152729840347416,
2.15472545757722));
#26096=CARTESIAN_POINT('Ctrl Pts',(0.631071654499439,-0.0197416511794313,
2.15457601125739));
#26097=CARTESIAN_POINT('Ctrl Pts',(0.629956339786456,-0.039290059680257,
2.157295074489));
#26098=CARTESIAN_POINT('Ctrl Pts',(0.628841025073472,-0.0578960018528886,
2.16305730877361));
#26099=CARTESIAN_POINT('Ctrl Pts',(0.625189679704009,-0.118808603476159,
2.1819218563564));
#26100=CARTESIAN_POINT('Ctrl Pts',(0.621538334334546,-0.169619915851716,
2.23340290186278));
#26101=CARTESIAN_POINT('Ctrl Pts',(0.617886988965082,-0.187685029649559,
2.29455741289086));
#26102=CARTESIAN_POINT('Ctrl Pts',(0.614235643595619,-0.205750143447401,
2.35571192391893));
#26103=CARTESIAN_POINT('Ctrl Pts',(0.610584298226155,-0.191069058667529,
2.42653990046871));
#26104=CARTESIAN_POINT('Ctrl Pts',(0.606932952856692,-0.15018483214835,
2.47547534853885));
#26105=CARTESIAN_POINT('Ctrl Pts',(0.603281607487229,-0.10930060562917,
2.524410796609));
#26106=CARTESIAN_POINT('Ctrl Pts',(0.599630262117766,-0.0422132373706839,
2.55145371619953));
#26107=CARTESIAN_POINT('Ctrl Pts',(0.595978916748303,0.0211792443787588,
2.54455298193631));
#26108=CARTESIAN_POINT('Ctrl Pts',(0.59232757137884,0.0845717261282007,
2.53765224767309));
#26109=CARTESIAN_POINT('Ctrl Pts',(0.588676226009376,0.144269321368599,
2.49680785955613));
#26110=CARTESIAN_POINT('Ctrl Pts',(0.585024880639913,0.173666080429868,
2.44022084897972));
#26111=CARTESIAN_POINT('Ctrl Pts',(0.581373535270449,0.203062839491137,
2.38363383840331));
#26112=CARTESIAN_POINT('Ctrl Pts',(0.577722189900986,0.202158762373277,
2.31130420536744));
#26113=CARTESIAN_POINT('Ctrl Pts',(0.574070844531523,0.171358441495245,
2.25547037582024));
#26114=CARTESIAN_POINT('Ctrl Pts',(0.57041949916206,0.140558120617212,2.19963654627303));
#26115=CARTESIAN_POINT('Ctrl Pts',(0.566768153792596,0.0798615559790066,
2.16029852021448));
#26116=CARTESIAN_POINT('Ctrl Pts',(0.563116808423133,0.0163157428736723,
2.1549806077331));
#26117=CARTESIAN_POINT('Ctrl Pts',(0.562806862019563,0.0109216225588305,
2.15452919388934));
#26118=CARTESIAN_POINT('Ctrl Pts',(0.562496915615993,0.00550697183036078,
2.15432291381032));
#26119=CARTESIAN_POINT('Ctrl Pts',(0.562186969212423,8.98932785041182E-5,
2.15435395233057));
#26120=CARTESIAN_POINT('Origin',(1.05400562256037,0.,2.35));
#26121=CARTESIAN_POINT('',(0.52900562256037,9.51678377910506E-5,2.19429007075223));
#26122=CARTESIAN_POINT('',(0.5204,-2.14950933638427E-15,2.19445));
#26123=CARTESIAN_POINT('',(1.05400562256037,-2.14950933638427E-15,2.19445));
#26124=CARTESIAN_POINT('',(0.5204,-0.108754917490551,2.23849675560759));
#26125=CARTESIAN_POINT('Ctrl Pts',(0.52900562256037,9.51678377910398E-5,
2.19429007075223));
#26126=CARTESIAN_POINT('Ctrl Pts',(0.526137081706913,-0.0398444327547342,
2.19455680225596));
#26127=CARTESIAN_POINT('Ctrl Pts',(0.523268540853457,-0.0799926191159976,
2.21081160130798));
#26128=CARTESIAN_POINT('Ctrl Pts',(0.5204,-0.108759141326515,2.23849470445504));
#26129=CARTESIAN_POINT('Origin',(0.5204,0.,2.35));
#26130=CARTESIAN_POINT('Origin',(1.05400562256037,0.,2.35));
#26131=CARTESIAN_POINT('',(0.59900562256037,-0.000128570015209672,2.19451094833158));
#26132=CARTESIAN_POINT('',(0.58519437743963,7.15603862352279E-5,2.19425413144842));
#26133=CARTESIAN_POINT('',(1.05400562256037,-2.14950933638427E-15,2.19445));
#26134=CARTESIAN_POINT('Ctrl Pts',(0.59900562256037,-0.000128570015209668,
2.19451094833158));
#26135=CARTESIAN_POINT('Ctrl Pts',(0.597996720623014,-0.0142256572937251,
2.19439471562695));
#26136=CARTESIAN_POINT('Ctrl Pts',(0.593336473316195,-0.0792100279504878,
2.20254628731932));
#26137=CARTESIAN_POINT('Ctrl Pts',(0.585024880639913,-0.173920106812228,
2.29315620321465));
#26138=CARTESIAN_POINT('Ctrl Pts',(0.574070844531523,-0.143717013770999,
2.46324494484324));
#26139=CARTESIAN_POINT('Ctrl Pts',(0.563116808423133,0.014578095564083,
2.53238460543625));
#26140=CARTESIAN_POINT('Ctrl Pts',(0.552162772314743,0.159893398509083,
2.43898045182826));
#26141=CARTESIAN_POINT('Ctrl Pts',(0.541208736206353,0.162663291181281,
2.2662242161504));
#26142=CARTESIAN_POINT('Ctrl Pts',(0.533489686288229,0.0624852719175517,
2.19716384358485));
#26143=CARTESIAN_POINT('Ctrl Pts',(0.529421981739568,0.00589226823472279,
2.19425135556021));
#26144=CARTESIAN_POINT('Ctrl Pts',(0.52900562256037,9.51678377910398E-5,
2.19429007075223));
#26145=CARTESIAN_POINT('',(0.5204,0.0700655924093113,2.21112374119263));
#26146=CARTESIAN_POINT('Origin',(0.5204,0.,2.35));
#26147=CARTESIAN_POINT('Ctrl Pts',(0.58519437743963,7.15603862352183E-5,
2.19425413144842));
#26148=CARTESIAN_POINT('Ctrl Pts',(0.581852978473736,-0.046417666264194,
2.19452050321855));
#26149=CARTESIAN_POINT('Ctrl Pts',(0.574860234138379,-0.144178508701954,
2.24102737311269));
#26150=CARTESIAN_POINT('Ctrl Pts',(0.56421614443356,-0.174115819489472,
2.40622641443997));
#26151=CARTESIAN_POINT('Ctrl Pts',(0.55326210832517,-0.0497712388056558,
2.52603005943954));
#26152=CARTESIAN_POINT('Ctrl Pts',(0.54230807221678,0.119016533293403,2.48911101549988));
#26153=CARTESIAN_POINT('Ctrl Pts',(0.53135403610839,0.181561589671221,2.32783318660189));
#26154=CARTESIAN_POINT('Ctrl Pts',(0.524051345369463,0.115581452136368,
2.23408731828768));
#26155=CARTESIAN_POINT('Ctrl Pts',(0.5204,0.0700655924093113,2.21112374119263));
#26156=CARTESIAN_POINT('Origin',(1.05400562256037,0.,2.35));
#26157=CARTESIAN_POINT('',(0.66900562256037,0.000111201918452189,2.19458402994267));
#26158=CARTESIAN_POINT('',(0.655194377439629,-0.000121582019789068,2.19454987167931));
#26159=CARTESIAN_POINT('',(1.05400562256037,-2.14950933638427E-15,2.19445));
#26160=CARTESIAN_POINT('Ctrl Pts',(0.66900562256037,0.0001112019184522,
2.19458402994267));
#26161=CARTESIAN_POINT('Ctrl Pts',(0.666571459506461,-0.0339414367351281,
2.19481764915658));
#26162=CARTESIAN_POINT('Ctrl Pts',(0.660485951083088,-0.11941940134295,
2.22244401000061));
#26163=CARTESIAN_POINT('Ctrl Pts',(0.650749097290252,-0.182550726710429,
2.36241526987937));
#26164=CARTESIAN_POINT('Ctrl Pts',(0.639795061181862,-0.0908611363653908,
2.5088180240845));
#26165=CARTESIAN_POINT('Ctrl Pts',(0.628841025073472,0.0818155011832931,
2.51366148576568));
#26166=CARTESIAN_POINT('Ctrl Pts',(0.617886988965083,0.181567845985935,
2.37262906836985));
#26167=CARTESIAN_POINT('Ctrl Pts',(0.607941854794048,0.125201242106021,
2.22627332924704));
#26168=CARTESIAN_POINT('Ctrl Pts',(0.601648065992477,0.0367935076532955,
2.19481537667645));
#26169=CARTESIAN_POINT('Ctrl Pts',(0.59900562256037,-0.000128570015209668,
2.19451094833158));
#26170=CARTESIAN_POINT('Ctrl Pts',(0.655194377439629,-0.000121582019789061,
2.19454987167931));
#26171=CARTESIAN_POINT('Ctrl Pts',(0.654079062726646,-0.0157155263099339,
2.19443090353678));
#26172=CARTESIAN_POINT('Ctrl Pts',(0.649312402644199,-0.082223484242051,
2.20368175088914));
#26173=CARTESIAN_POINT('Ctrl Pts',(0.640894397192289,-0.175476343657893,
2.29816375646506));
#26174=CARTESIAN_POINT('Ctrl Pts',(0.629940361083899,-0.140415298557959,
2.46731357866031));
#26175=CARTESIAN_POINT('Ctrl Pts',(0.618986324975509,0.0198012848495282,
2.53189688688404));
#26176=CARTESIAN_POINT('Ctrl Pts',(0.60803228886712,0.16236977419923,2.4343532138299));
#26177=CARTESIAN_POINT('Ctrl Pts',(0.597078252758729,0.160210677029069,
2.26161716850653));
#26178=CARTESIAN_POINT('Ctrl Pts',(0.589465615616233,0.0594730344796908,
2.19632813557188));
#26179=CARTESIAN_POINT('Ctrl Pts',(0.5855043238432,0.00438387650057295,
2.19422942294368));
#26180=CARTESIAN_POINT('Ctrl Pts',(0.58519437743963,7.15603862352183E-5,
2.19425413144842));
#26181=CARTESIAN_POINT('Origin',(1.05400562256037,0.,2.35));
#26182=CARTESIAN_POINT('',(0.73900562256037,-4.93584221261508E-5,2.19422991105133));
#26183=CARTESIAN_POINT('',(0.725194377439629,0.000121981686909765,2.19454823264579));
#26184=CARTESIAN_POINT('',(1.05400562256037,-2.14950933638427E-15,2.19445));
#26185=CARTESIAN_POINT('Ctrl Pts',(0.73900562256037,-4.93584221261476E-5,
2.19422991105133));
#26186=CARTESIAN_POINT('Ctrl Pts',(0.738797543759371,-0.00294318160930773,
2.19421764985331));
#26187=CARTESIAN_POINT('Ctrl Pts',(0.734938119588908,-0.0566056877646526,
2.19558775087244));
#26188=CARTESIAN_POINT('Ctrl Pts',(0.727427350048981,-0.157727895671703,
2.2572594409398));
#26189=CARTESIAN_POINT('Ctrl Pts',(0.716473313940592,-0.164621520822112,
2.42986649077344));
#26190=CARTESIAN_POINT('Ctrl Pts',(0.705519277832201,-0.0247832025340387,
2.53128622214169));
#26191=CARTESIAN_POINT('Ctrl Pts',(0.694565241723812,0.137145099584703,
2.47112027917621));
#26192=CARTESIAN_POINT('Ctrl Pts',(0.683611205615422,0.176831999341087,
2.30299632262599));
#26193=CARTESIAN_POINT('Ctrl Pts',(0.675091332560941,0.0851090304351673,
2.20481803865857));
#26194=CARTESIAN_POINT('Ctrl Pts',(0.670222804875924,0.0171389312238162,
2.19446721066252));
#26195=CARTESIAN_POINT('Ctrl Pts',(0.66900562256037,0.0001112019184522,
2.19458402994267));
#26196=CARTESIAN_POINT('Ctrl Pts',(0.725194377439629,0.000121981686909774,
2.19454823264579));
#26197=CARTESIAN_POINT('Ctrl Pts',(0.722653801610092,-0.035398541373101,
2.19482031234125));
#26198=CARTESIAN_POINT('Ctrl Pts',(0.716461880411091,-0.122379100748218,
2.22436899345466));
#26199=CARTESIAN_POINT('Ctrl Pts',(0.706618613842629,-0.182120023079803,
2.36764042281014));
#26200=CARTESIAN_POINT('Ctrl Pts',(0.695664577734238,-0.086273578795776,
2.51135599819781));
#26201=CARTESIAN_POINT('Ctrl Pts',(0.684710541625849,0.0864709980175075,
2.51125026394776));
#26202=CARTESIAN_POINT('Ctrl Pts',(0.673756505517459,0.182141488128614,
2.36741754065941));
#26203=CARTESIAN_POINT('Ctrl Pts',(0.663917784122053,0.122252892767114,
2.22428537964787));
#26204=CARTESIAN_POINT('Ctrl Pts',(0.657730408096109,0.0353363208616827,
2.19482038443511));
#26205=CARTESIAN_POINT('Ctrl Pts',(0.655194377439629,-0.000121582019789061,
2.19454987167931));
#26206=CARTESIAN_POINT('Origin',(1.05400562256037,0.,2.35));
#26207=CARTESIAN_POINT('',(0.80900562256037,-4.08630748678726E-5,2.19467648483088));
#26208=CARTESIAN_POINT('',(0.79519437743963,-7.19606880817819E-5,2.19425418850934));
#26209=CARTESIAN_POINT('',(1.05400562256037,-2.14950933638427E-15,2.19445));
#26210=CARTESIAN_POINT('Ctrl Pts',(0.80900562256037,-4.08630748678709E-5,
2.19467648483088));
#26211=CARTESIAN_POINT('Ctrl Pts',(0.807372282642817,-0.02292474521305,
2.19462097806632));
#26212=CARTESIAN_POINT('Ctrl Pts',(0.802087597355801,-0.0968949254760526,
2.20997973041345));
#26213=CARTESIAN_POINT('Ctrl Pts',(0.793151566699321,-0.180979052586637,
2.32306599395291));
#26214=CARTESIAN_POINT('Ctrl Pts',(0.782197530590931,-0.12274025290824,
2.48569724091423));
#26215=CARTESIAN_POINT('Ctrl Pts',(0.771243494482541,0.0449007034323279,
2.52737765806314));
#26216=CARTESIAN_POINT('Ctrl Pts',(0.760289458374152,0.172520254747402,
2.41095619106118));
#26217=CARTESIAN_POINT('Ctrl Pts',(0.74954350106676,0.146864336702308,2.24344628678707));
#26218=CARTESIAN_POINT('Ctrl Pts',(0.742448889128834,0.0478373296383567,
2.19443280809342));
#26219=CARTESIAN_POINT('Ctrl Pts',(0.73900562256037,-4.93584221261476E-5,
2.19422991105133));
#26220=CARTESIAN_POINT('Ctrl Pts',(0.79519437743963,-7.19606880817871E-5,
2.19425418850934));
#26221=CARTESIAN_POINT('Ctrl Pts',(0.794879885863002,-0.00444751424563119,
2.19422865519439));
#26222=CARTESIAN_POINT('Ctrl Pts',(0.790914048916912,-0.0595994116820262,
2.19635851179074));
#26223=CARTESIAN_POINT('Ctrl Pts',(0.783296866601358,-0.160320194189603,
2.26181657493399));
#26224=CARTESIAN_POINT('Ctrl Pts',(0.772342830492968,-0.16226566916103,
2.43455022864764));
#26225=CARTESIAN_POINT('Ctrl Pts',(0.761388794384578,-0.0195790184948705,
2.53192182210578));
#26226=CARTESIAN_POINT('Ctrl Pts',(0.750434758276188,0.140558966382812,
2.46714120953931));
#26227=CARTESIAN_POINT('Ctrl Pts',(0.739480722167798,0.175412672397597,
2.29794924135903));
#26228=CARTESIAN_POINT('Ctrl Pts',(0.731067261888946,0.0820947684486603,
2.20363214347216));
#26229=CARTESIAN_POINT('Ctrl Pts',(0.726305146979556,0.0156519708329137,
2.19442927621291));
#26230=CARTESIAN_POINT('Ctrl Pts',(0.725194377439629,0.000121981686909774,
2.19454823264579));
#26231=CARTESIAN_POINT('Origin',(1.05400562256037,0.,2.35));
#26232=CARTESIAN_POINT('',(0.87900562256037,0.000124190176919192,2.19434837072514));
#26233=CARTESIAN_POINT('',(0.865194377439629,-1.79285551041297E-5,2.1946855147081));
#26234=CARTESIAN_POINT('',(1.05400562256037,-2.14950933638427E-15,2.19445));
#26235=CARTESIAN_POINT('Ctrl Pts',(0.87900562256037,0.000124190176919186,
2.19434837072514));
#26236=CARTESIAN_POINT('Ctrl Pts',(0.875947021526264,-0.0424956765806325,
2.19470411582899));
#26237=CARTESIAN_POINT('Ctrl Pts',(0.869237075122694,-0.136605475911018,
2.23469767016882));
#26238=CARTESIAN_POINT('Ctrl Pts',(0.858875783349661,-0.177891546494684,
2.39279325713406));
#26239=CARTESIAN_POINT('Ctrl Pts',(0.847921747241271,-0.0630038111484079,
2.52178334424669));
#26240=CARTESIAN_POINT('Ctrl Pts',(0.83696771113288,0.108053315947243,2.49766144283244));
#26241=CARTESIAN_POINT('Ctrl Pts',(0.826013675024491,0.18279317314933,2.34192284359958));
#26242=CARTESIAN_POINT('Ctrl Pts',(0.816692978833654,0.107756578718704,
2.21553286752609));
#26243=CARTESIAN_POINT('Ctrl Pts',(0.81102362801228,0.028232369226284,2.19474506391372));
#26244=CARTESIAN_POINT('Ctrl Pts',(0.80900562256037,-4.08630748678709E-5,
2.19467648483088));
#26245=CARTESIAN_POINT('Ctrl Pts',(0.865194377439629,-1.79285551041419E-5,
2.19468551470809));
#26246=CARTESIAN_POINT('Ctrl Pts',(0.863454624746448,-0.0243964419532612,
2.19465869077632));
#26247=CARTESIAN_POINT('Ctrl Pts',(0.858063526683804,-0.0999055619129348,
2.21143804034893));
#26248=CARTESIAN_POINT('Ctrl Pts',(0.849021083251698,-0.181675685171884,
2.32826261843907));
#26249=CARTESIAN_POINT('Ctrl Pts',(0.838067047143307,-0.118802362076862,
2.48915793391742));
#26250=CARTESIAN_POINT('Ctrl Pts',(0.827113011034918,0.0499644633958529,
2.52601845279664));
#26251=CARTESIAN_POINT('Ctrl Pts',(0.816158974926527,0.174195747659866,
2.40598825754555));
#26252=CARTESIAN_POINT('Ctrl Pts',(0.805519430394765,0.14405268557978,2.24093310845852));
#26253=CARTESIAN_POINT('Ctrl Pts',(0.798531231232466,0.0463540283347385,
2.19452510495093));
#26254=CARTESIAN_POINT('Ctrl Pts',(0.79519437743963,-7.19606880817871E-5,
2.19425418850934));
#26255=CARTESIAN_POINT('Origin',(0.5204,-2.59090492670967E-17,2.35));
#26256=CARTESIAN_POINT('',(0.5204,-0.0584934195161147,2.53643948045763));
#26257=CARTESIAN_POINT('Ctrl Pts',(0.5204,-0.108759141326515,2.23849470445504));
#26258=CARTESIAN_POINT('Ctrl Pts',(0.5204,-0.112907330059273,2.24159827661415));
#26259=CARTESIAN_POINT('Ctrl Pts',(0.5204,-0.116881232068949,2.24491115539772));
#26260=CARTESIAN_POINT('Ctrl Pts',(0.5204,-0.120661377643655,2.24842558763538));
#26261=CARTESIAN_POINT('Ctrl Pts',(0.5204,-0.125564505420802,2.2529840656053));
#26262=CARTESIAN_POINT('Ctrl Pts',(0.5204,-0.130141932979661,2.25788137180214));
#26263=CARTESIAN_POINT('Ctrl Pts',(0.5204,-0.134389577775584,2.26307215460619));
#26264=CARTESIAN_POINT('Ctrl Pts',(0.5204,-0.137535387529399,2.26691645326096));
#26265=CARTESIAN_POINT('Ctrl Pts',(0.5204,-0.140500968847107,2.27092391847997));
#26266=CARTESIAN_POINT('Ctrl Pts',(0.5204,-0.143271491547599,2.27505836426546));
#26267=CARTESIAN_POINT('Ctrl Pts',(0.5204,-0.148395262305637,2.28270455767603));
#26268=CARTESIAN_POINT('Ctrl Pts',(0.5204,-0.15286388444708,2.29079619664306));
#26269=CARTESIAN_POINT('Ctrl Pts',(0.5204,-0.156663462872097,2.29922509487536));
#26270=CARTESIAN_POINT('Ctrl Pts',(0.5204,-0.158675814066677,2.30368924892863));
#26271=CARTESIAN_POINT('Ctrl Pts',(0.5204,-0.160500911014214,2.30825162957441));
#26272=CARTESIAN_POINT('Ctrl Pts',(0.5204,-0.162127268087927,2.31287264211295));
#26273=CARTESIAN_POINT('Ctrl Pts',(0.5204,-0.166006645959223,2.32389522385391));
#26274=CARTESIAN_POINT('Ctrl Pts',(0.5204,-0.168771336018711,2.33527453234392));
#26275=CARTESIAN_POINT('Ctrl Pts',(0.5204,-0.170389890260227,2.34680888322882));
#26276=CARTESIAN_POINT('Ctrl Pts',(0.5204,-0.171128381708844,2.35207161664569));
#26277=CARTESIAN_POINT('Ctrl Pts',(0.5204,-0.171627714504877,2.35736710228387));
#26278=CARTESIAN_POINT('Ctrl Pts',(0.5204,-0.171881743379811,2.36267782474742));
#26279=CARTESIAN_POINT('Ctrl Pts',(0.5204,-0.172104849855246,2.36734208415953));
#26280=CARTESIAN_POINT('Ctrl Pts',(0.5204,-0.172138134548399,2.37202236286416));
#26281=CARTESIAN_POINT('Ctrl Pts',(0.5204,-0.17197823645371,2.37667856889389));
#26282=CARTESIAN_POINT('Ctrl Pts',(0.5204,-0.171715082631453,2.38434156460574));
#26283=CARTESIAN_POINT('Ctrl Pts',(0.5204,-0.170930692380004,2.39195277755355));
#26284=CARTESIAN_POINT('Ctrl Pts',(0.5204,-0.169614423041612,2.39945925007218));
#26285=CARTESIAN_POINT('Ctrl Pts',(0.5204,-0.168268512776876,2.40713476003059));
#26286=CARTESIAN_POINT('Ctrl Pts',(0.5204,-0.166366695988795,2.41470100550351));
#26287=CARTESIAN_POINT('Ctrl Pts',(0.5204,-0.163950619192884,2.42212362412655));
#26288=CARTESIAN_POINT('Ctrl Pts',(0.5204,-0.162575528939075,2.42634814651903));
#26289=CARTESIAN_POINT('Ctrl Pts',(0.5204,-0.161033657153843,2.43052615011737));
#26290=CARTESIAN_POINT('Ctrl Pts',(0.5204,-0.159331206362488,2.43465111681409));
#26291=CARTESIAN_POINT('Ctrl Pts',(0.5204,-0.157858857773026,2.43821855554908));
#26292=CARTESIAN_POINT('Ctrl Pts',(0.5204,-0.156269236378672,2.44173904368652));
#26293=CARTESIAN_POINT('Ctrl Pts',(0.5204,-0.154570626304257,2.44520268317124));
#26294=CARTESIAN_POINT('Ctrl Pts',(0.5204,-0.149623492625337,2.45529039417953));
#26295=CARTESIAN_POINT('Ctrl Pts',(0.5204,-0.143748121077635,2.46491226866532));
#26296=CARTESIAN_POINT('Ctrl Pts',(0.5204,-0.137061858098255,2.47397051071086));
#26297=CARTESIAN_POINT('Ctrl Pts',(0.5204,-0.132163446938004,2.48060665321153));
#26298=CARTESIAN_POINT('Ctrl Pts',(0.5204,-0.126828911752323,2.48694038241048));
#26299=CARTESIAN_POINT('Ctrl Pts',(0.5204,-0.121092850543412,2.49292921348278));
#26300=CARTESIAN_POINT('Ctrl Pts',(0.5204,-0.118821952815951,2.49530018240674));
#26301=CARTESIAN_POINT('Ctrl Pts',(0.5204,-0.116489100525108,2.49761568017534));
#26302=CARTESIAN_POINT('Ctrl Pts',(0.5204,-0.114103581939124,2.49986675461349));
#26303=CARTESIAN_POINT('Ctrl Pts',(0.5204,-0.10477538102635,2.5086692325116));
#26304=CARTESIAN_POINT('Ctrl Pts',(0.5204,-0.0946182126828188,2.51651747522707));
#26305=CARTESIAN_POINT('Ctrl Pts',(0.5204,-0.0837748677305257,2.52326941089188));
#26306=CARTESIAN_POINT('Ctrl Pts',(0.5204,-0.0757132037363705,2.52828924903955));
#26307=CARTESIAN_POINT('Ctrl Pts',(0.5204,-0.0672710749325205,2.53270298831844));
#26308=CARTESIAN_POINT('Ctrl Pts',(0.5204,-0.058493419516116,2.53643948045763));
#26309=CARTESIAN_POINT('',(0.5204,-2.39295984553393E-17,2.1546));
#26310=CARTESIAN_POINT('Origin',(0.5204,0.,2.35));
#26311=CARTESIAN_POINT('',(0.5204,0.112041393629813,2.51041297594259));
#26312=CARTESIAN_POINT('Origin',(0.5204,0.,2.35));
#26313=CARTESIAN_POINT('Ctrl Pts',(0.5204,0.112041393629812,2.51041297594259));
#26314=CARTESIAN_POINT('Ctrl Pts',(0.5204,0.116937045114913,2.50627340682946));
#26315=CARTESIAN_POINT('Ctrl Pts',(0.5204,0.121606025691287,2.50188933924213));
#26316=CARTESIAN_POINT('Ctrl Pts',(0.5204,0.1260235014566,2.49726406054717));
#26317=CARTESIAN_POINT('Ctrl Pts',(0.5204,0.132755493122292,2.49021538857244));
#26318=CARTESIAN_POINT('Ctrl Pts',(0.5204,0.138904187281487,2.48260660874921));
#26319=CARTESIAN_POINT('Ctrl Pts',(0.5204,0.144439872512489,2.47452670862429));
#26320=CARTESIAN_POINT('Ctrl Pts',(0.5204,0.146734801839087,2.47117702399107));
#26321=CARTESIAN_POINT('Ctrl Pts',(0.5204,0.148922511137616,2.46774842779565));
#26322=CARTESIAN_POINT('Ctrl Pts',(0.5204,0.150996712083198,2.46425475963724));
#26323=CARTESIAN_POINT('Ctrl Pts',(0.5204,0.154797431035443,2.45785304103288));
#26324=CARTESIAN_POINT('Ctrl Pts',(0.5204,0.158222183852141,2.45122603720417));
#26325=CARTESIAN_POINT('Ctrl Pts',(0.5204,0.161257886649128,2.44441406179352));
#26326=CARTESIAN_POINT('Ctrl Pts',(0.5204,0.163547894840152,2.43927539027964));
#26327=CARTESIAN_POINT('Ctrl Pts',(0.5204,0.165616393075825,2.43403139932254));
#26328=CARTESIAN_POINT('Ctrl Pts',(0.5204,0.167455419852478,2.42869927944118));
#26329=CARTESIAN_POINT('Ctrl Pts',(0.5204,0.1688297887935,2.42471440002139));
#26330=CARTESIAN_POINT('Ctrl Pts',(0.5204,0.1700730662053,2.42068834043065));
#26331=CARTESIAN_POINT('Ctrl Pts',(0.5204,0.171181794352447,2.41663368257067));
#26332=CARTESIAN_POINT('Ctrl Pts',(0.5204,0.174401260833582,2.40485998032791));
#26333=CARTESIAN_POINT('Ctrl Pts',(0.5204,0.176494813205288,2.39283081517787));
#26334=CARTESIAN_POINT('Ctrl Pts',(0.5204,0.177388397835593,2.38072640253141));
#26335=CARTESIAN_POINT('Ctrl Pts',(0.5204,0.177810038893935,2.37501489274734));
#26336=CARTESIAN_POINT('Ctrl Pts',(0.5204,0.177963781655902,2.36928669844613));
#26337=CARTESIAN_POINT('Ctrl Pts',(0.5204,0.177837820477668,2.36356196196988));
#26338=CARTESIAN_POINT('Ctrl Pts',(0.5204,0.177744132474277,2.35930399028433));
#26339=CARTESIAN_POINT('Ctrl Pts',(0.5204,0.177495088766334,2.35504632454376));
#26340=CARTESIAN_POINT('Ctrl Pts',(0.5204,0.177088122483941,2.35081883251768));
#26341=CARTESIAN_POINT('Ctrl Pts',(0.5204,0.176379013755951,2.34345273949499));
#26342=CARTESIAN_POINT('Ctrl Pts',(0.5204,0.175191118127969,2.33616306535315));
#26343=CARTESIAN_POINT('Ctrl Pts',(0.5204,0.173504620809491,2.32899257319754));
#26344=CARTESIAN_POINT('Ctrl Pts',(0.5204,0.17195948112857,2.32242309227399));
#26345=CARTESIAN_POINT('Ctrl Pts',(0.5204,0.169995611849258,2.31595359739138));
#26346=CARTESIAN_POINT('Ctrl Pts',(0.5204,0.167635724455005,2.30961315508381));
#26347=CARTESIAN_POINT('Ctrl Pts',(0.5204,0.165837815689064,2.30478261239246));
#26348=CARTESIAN_POINT('Ctrl Pts',(0.5204,0.163809931535238,2.3000270249417));
#26349=CARTESIAN_POINT('Ctrl Pts',(0.5204,0.161560656715894,2.29536084562219));
#26350=CARTESIAN_POINT('Ctrl Pts',(0.5204,0.160071713441668,2.29227199393792));
#26351=CARTESIAN_POINT('Ctrl Pts',(0.5204,0.158487800659087,2.28922696718331));
#26352=CARTESIAN_POINT('Ctrl Pts',(0.5204,0.156815851991927,2.28623595701929));
#26353=CARTESIAN_POINT('Ctrl Pts',(0.5204,0.152047341533174,2.27770539413208));
#26354=CARTESIAN_POINT('Ctrl Pts',(0.5204,0.14655595542121,2.26959575714595));
#26355=CARTESIAN_POINT('Ctrl Pts',(0.5204,0.140413115121167,2.26199694931317));
#26356=CARTESIAN_POINT('Ctrl Pts',(0.5204,0.136686501207848,2.25738705851167));
#26357=CARTESIAN_POINT('Ctrl Pts',(0.5204,0.132719734840018,2.25296552232463));
#26358=CARTESIAN_POINT('Ctrl Pts',(0.5204,0.128526293595978,2.24875666671166));
#26359=CARTESIAN_POINT('Ctrl Pts',(0.5204,0.12615221987615,2.24637386630507));
#26360=CARTESIAN_POINT('Ctrl Pts',(0.5204,0.123703674799012,2.24405772039151));
#26361=CARTESIAN_POINT('Ctrl Pts',(0.5204,0.121188860554935,2.24181840024681));
#26362=CARTESIAN_POINT('Ctrl Pts',(0.5204,0.113088816925757,2.23460570415423));
#26363=CARTESIAN_POINT('Ctrl Pts',(0.5204,0.104340638126238,2.22821818956216));
#26364=CARTESIAN_POINT('Ctrl Pts',(0.5204,0.095037049653237,2.22279264290421));
#26365=CARTESIAN_POINT('Ctrl Pts',(0.5204,0.0871009281534262,2.21816455798781));
#26366=CARTESIAN_POINT('Ctrl Pts',(0.5204,0.0787597846219885,2.2142367405948));
#26367=CARTESIAN_POINT('Ctrl Pts',(0.5204,0.0700655924093113,2.21112374119263));
#26368=CARTESIAN_POINT('Ctrl Pts',(0.947607408227206,0.139614588036676,
2.28141742708713));
#26369=CARTESIAN_POINT('Ctrl Pts',(0.943956062857743,0.117137061674501,
2.23565958438961));
#26370=CARTESIAN_POINT('Ctrl Pts',(0.936653372118816,0.0240992050028806,
2.16868478613642));
#26371=CARTESIAN_POINT('Ctrl Pts',(0.925699336010427,-0.13783558819615,
2.22950867061399));
#26372=CARTESIAN_POINT('Ctrl Pts',(0.914745299902037,-0.17655014467161,
2.39789367865357));
#26373=CARTESIAN_POINT('Ctrl Pts',(0.903791263793647,-0.0580775762076774,
2.52350712786254));
#26374=CARTESIAN_POINT('Ctrl Pts',(0.892837227685257,0.112250391536416,
2.49451043435059));
#26375=CARTESIAN_POINT('Ctrl Pts',(0.881883191576867,0.182481185996413,
2.33668621664117));
#26376=CARTESIAN_POINT('Ctrl Pts',(0.870929155468477,0.09008407841159,2.19073969498444));
#26377=CARTESIAN_POINT('Ctrl Pts',(0.859975119360086,-0.0826191757791262,
2.18674106440834));
#26378=CARTESIAN_POINT('Ctrl Pts',(0.849021083251698,-0.181675685171884,
2.32826261843907));
#26379=CARTESIAN_POINT('Ctrl Pts',(0.838067047143307,-0.118802362076862,
2.48915793391742));
#26380=CARTESIAN_POINT('Ctrl Pts',(0.827113011034918,0.0499644633958529,
2.52601845279664));
#26381=CARTESIAN_POINT('Ctrl Pts',(0.816158974926527,0.174195747659866,
2.40598825754555));
#26382=CARTESIAN_POINT('Ctrl Pts',(0.805204938818138,0.14316169451436,2.23605428550592));
#26383=CARTESIAN_POINT('Ctrl Pts',(0.794250902709748,-0.0154767280957943,
2.16768334330683));
#26384=CARTESIAN_POINT('Ctrl Pts',(0.783296866601358,-0.160320194189603,
2.26181657493399));
#26385=CARTESIAN_POINT('Ctrl Pts',(0.772342830492968,-0.16226566916103,
2.43455022864764));
#26386=CARTESIAN_POINT('Ctrl Pts',(0.761388794384578,-0.0195790184948705,
2.53192182210578));
#26387=CARTESIAN_POINT('Ctrl Pts',(0.750434758276188,0.140558966382812,
2.46714120953931));
#26388=CARTESIAN_POINT('Ctrl Pts',(0.739480722167798,0.175412672397597,
2.29794924135903));
#26389=CARTESIAN_POINT('Ctrl Pts',(0.728526686059409,0.0539159688373249,
2.17515162163435));
#26390=CARTESIAN_POINT('Ctrl Pts',(0.717572649951018,-0.115637599199776,
2.20820143987244));
#26391=CARTESIAN_POINT('Ctrl Pts',(0.706618613842629,-0.182120023079803,
2.36764042281014));
#26392=CARTESIAN_POINT('Ctrl Pts',(0.695664577734238,-0.086273578795776,
2.51135599819781));
#26393=CARTESIAN_POINT('Ctrl Pts',(0.684710541625849,0.0864709980175075,
2.51125026394776));
#26394=CARTESIAN_POINT('Ctrl Pts',(0.673756505517459,0.182141488128614,
2.36741754065941));
#26395=CARTESIAN_POINT('Ctrl Pts',(0.662802469409069,0.115463938302179,
2.20805995780069));
#26396=CARTESIAN_POINT('Ctrl Pts',(0.651848433300678,-0.0541298804027574,
2.17521785121658));
#26397=CARTESIAN_POINT('Ctrl Pts',(0.640894397192289,-0.175476343657893,
2.29816375646506));
#26398=CARTESIAN_POINT('Ctrl Pts',(0.629940361083899,-0.140415298557959,
2.46731357866031));
#26399=CARTESIAN_POINT('Ctrl Pts',(0.618986324975509,0.0198012848495282,
2.53189688688404));
#26400=CARTESIAN_POINT('Ctrl Pts',(0.60803228886712,0.16236977419923,2.4343532138299));
#26401=CARTESIAN_POINT('Ctrl Pts',(0.597078252758729,0.160210677029069,
2.26161716850653));
#26402=CARTESIAN_POINT('Ctrl Pts',(0.58612421665034,0.0152564708447366,
2.16767095632525));
#26403=CARTESIAN_POINT('Ctrl Pts',(0.575170180541949,-0.143306760899327,
2.23621692429532));
#26404=CARTESIAN_POINT('Ctrl Pts',(0.56421614443356,-0.174115819489472,
2.40622641443997));
#26405=CARTESIAN_POINT('Ctrl Pts',(0.55326210832517,-0.0497712388056558,
2.52603005943954));
#26406=CARTESIAN_POINT('Ctrl Pts',(0.54230807221678,0.119016533293403,2.48911101549988));
#26407=CARTESIAN_POINT('Ctrl Pts',(0.53135403610839,0.181561589671221,2.32783318660189));
#26408=CARTESIAN_POINT('Ctrl Pts',(0.524051345369463,0.115581452136368,
2.23408731828768));
#26409=CARTESIAN_POINT('Ctrl Pts',(0.5204,0.0700655924093113,2.21112374119263));
#26410=CARTESIAN_POINT('Ctrl Pts',(0.939938272151471,0.151537102412036,
2.27556075606907));
#26411=CARTESIAN_POINT('Ctrl Pts',(0.936286926782008,0.127140087299121,
2.22589538089218));
#26412=CARTESIAN_POINT('Ctrl Pts',(0.928984236043081,0.0261571784720005,
2.15320120899624));
#26413=CARTESIAN_POINT('Ctrl Pts',(0.918030199934692,-0.14960618326658,
2.21921920425583));
#26414=CARTESIAN_POINT('Ctrl Pts',(0.907076163826301,-0.191626804406237,
2.4019836027816));
#26415=CARTESIAN_POINT('Ctrl Pts',(0.896122127717911,-0.0630371635041008,
2.53832392641675));
#26416=CARTESIAN_POINT('Ctrl Pts',(0.885168091609522,0.121836115532401,
2.50685103396244));
#26417=CARTESIAN_POINT('Ctrl Pts',(0.874214055501131,0.198064332384406,
2.33554927403568));
#26418=CARTESIAN_POINT('Ctrl Pts',(0.863260019392742,0.0977768899935077,
2.17713951678907));
#26419=CARTESIAN_POINT('Ctrl Pts',(0.852305983284352,-0.0896745152301024,
2.17279941952818));
#26420=CARTESIAN_POINT('Ctrl Pts',(0.841351947175961,-0.19719004508638,
2.32640633502494));
#26421=CARTESIAN_POINT('Ctrl Pts',(0.830397911067572,-0.128947597539763,
2.50104145190009));
#26422=CARTESIAN_POINT('Ctrl Pts',(0.819443874959181,0.0542312240651439,
2.54104970822135));
#26423=CARTESIAN_POINT('Ctrl Pts',(0.808489838850793,0.189071351526245,
2.41076942557982));
#26424=CARTESIAN_POINT('Ctrl Pts',(0.797535802742401,0.155387117264596,
2.22632378786831));
#26425=CARTESIAN_POINT('Ctrl Pts',(0.786581766634013,-0.0167983773288753,
2.15211424704791));
#26426=CARTESIAN_POINT('Ctrl Pts',(0.775627730525622,-0.174010882582308,
2.2542860713684));
#26427=CARTESIAN_POINT('Ctrl Pts',(0.764673694417233,-0.176122493153459,
2.44177047210978));
#26428=CARTESIAN_POINT('Ctrl Pts',(0.753719658308842,-0.0212509865373449,
2.54745720110699));
#26429=CARTESIAN_POINT('Ctrl Pts',(0.742765622200452,0.152562126803587,
2.47714458937461));
#26430=CARTESIAN_POINT('Ctrl Pts',(0.731811586092063,0.190392196655701,
2.29350431961502));
#26431=CARTESIAN_POINT('Ctrl Pts',(0.720857549983673,0.0585201718977931,
2.16022028577691));
#26432=CARTESIAN_POINT('Ctrl Pts',(0.709903513875282,-0.125512576866359,
2.19609242321952));
#26433=CARTESIAN_POINT('Ctrl Pts',(0.698949477766893,-0.197672327632959,
2.36914684271581));
#26434=CARTESIAN_POINT('Ctrl Pts',(0.687995441658503,-0.093640989306891,
2.52513514001327));
#26435=CARTESIAN_POINT('Ctrl Pts',(0.677041405550113,0.0938552673221205,
2.52502037649103));
#26436=CARTESIAN_POINT('Ctrl Pts',(0.666087369441724,0.197695625709081,
2.36890492734167));
#26437=CARTESIAN_POINT('Ctrl Pts',(0.655133333333334,0.125324086038902,
2.19593885915794));
#26438=CARTESIAN_POINT('Ctrl Pts',(0.644179297224943,-0.0587523506353723,
2.16029217109439));
#26439=CARTESIAN_POINT('Ctrl Pts',(0.633225261116554,-0.19046130518102,
2.2937371534331));
#26440=CARTESIAN_POINT('Ctrl Pts',(0.622271225008164,-0.152406190334525,
2.47733167811303));
#26441=CARTESIAN_POINT('Ctrl Pts',(0.611317188899773,0.021492233528953,
2.54743013651938));
#26442=CARTESIAN_POINT('Ctrl Pts',(0.600363152791384,0.176235488335819,
2.44155663303299));
#26443=CARTESIAN_POINT('Ctrl Pts',(0.589409116682993,0.173892013104519,
2.25406963644822));
#26444=CARTESIAN_POINT('Ctrl Pts',(0.578455080574605,0.0165593110100914,
2.15210080226881));
#26445=CARTESIAN_POINT('Ctrl Pts',(0.567501044466214,-0.155544571725081,
2.22650031534464));
#26446=CARTESIAN_POINT('Ctrl Pts',(0.556547008357824,-0.188984597817245,
2.41102792009824));
#26447=CARTESIAN_POINT('Ctrl Pts',(0.545592972249434,-0.0540214988858134,
2.54106230602406));
#26448=CARTESIAN_POINT('Ctrl Pts',(0.534638936141044,0.129180058101593,
2.50099052684172));
#26449=CARTESIAN_POINT('Ctrl Pts',(0.523684900032654,0.197066206296954,
2.32594023146654));
#26450=CARTESIAN_POINT('Ctrl Pts',(0.516382209293728,0.125451635073546,
2.22418884970044));
#26451=CARTESIAN_POINT('Ctrl Pts',(0.512730863924265,0.0760489072223641,
2.19926427711147));
#26452=CARTESIAN_POINT('Ctrl Pts',(0.932269136075735,0.163459616787395,
2.26970408505101));
#26453=CARTESIAN_POINT('Ctrl Pts',(0.928617790706272,0.137143112923741,
2.21613117739475));
#26454=CARTESIAN_POINT('Ctrl Pts',(0.921315099967345,0.0282151519411206,
2.13771763185606));
#26455=CARTESIAN_POINT('Ctrl Pts',(0.910361063858956,-0.161376778337011,
2.20892973789767));
#26456=CARTESIAN_POINT('Ctrl Pts',(0.899407027750565,-0.206703464140864,
2.40607352690963));
#26457=CARTESIAN_POINT('Ctrl Pts',(0.888452991642176,-0.0679967508005241,
2.55314072497096));
#26458=CARTESIAN_POINT('Ctrl Pts',(0.877498955533787,0.131421839528385,
2.5191916335743));
#26459=CARTESIAN_POINT('Ctrl Pts',(0.866544919425395,0.213647478772399,
2.3344123314302));
#26460=CARTESIAN_POINT('Ctrl Pts',(0.855590883317007,0.105469701575425,
2.16353933859369));
#26461=CARTESIAN_POINT('Ctrl Pts',(0.844636847208615,-0.0967298546810787,
2.15885777464802));
#26462=CARTESIAN_POINT('Ctrl Pts',(0.833682811100226,-0.212704405000876,
2.32455005161081));
#26463=CARTESIAN_POINT('Ctrl Pts',(0.822728774991836,-0.139092833002665,
2.51292496988275));
#26464=CARTESIAN_POINT('Ctrl Pts',(0.811774738883447,0.0584979847344349,
2.55608096364608));
#26465=CARTESIAN_POINT('Ctrl Pts',(0.800820702775056,0.203946955392624,
2.41555059361408));
#26466=CARTESIAN_POINT('Ctrl Pts',(0.789866666666667,0.167612540014831,
2.2165932902307));
#26467=CARTESIAN_POINT('Ctrl Pts',(0.778912630558277,-0.0181200265619565,
2.13654515078899));
#26468=CARTESIAN_POINT('Ctrl Pts',(0.767958594449887,-0.187701570975013,
2.24675556780282));
#26469=CARTESIAN_POINT('Ctrl Pts',(0.757004558341496,-0.189979317145888,
2.44899071557192));
#26470=CARTESIAN_POINT('Ctrl Pts',(0.746050522233108,-0.0229229545798194,
2.5629925801082));
#26471=CARTESIAN_POINT('Ctrl Pts',(0.735096486124716,0.164565287224363,
2.48714796920991));
#26472=CARTESIAN_POINT('Ctrl Pts',(0.724142450016328,0.205371720913805,
2.28905939787101));
#26473=CARTESIAN_POINT('Ctrl Pts',(0.713188413907937,0.0631243749582614,
2.14528894991948));
#26474=CARTESIAN_POINT('Ctrl Pts',(0.702234377799548,-0.135387554532942,
2.18398340656661));
#26475=CARTESIAN_POINT('Ctrl Pts',(0.691280341691157,-0.213224632186115,
2.37065326262149));
#26476=CARTESIAN_POINT('Ctrl Pts',(0.680326305582768,-0.101008399818006,
2.53891428182873));
#26477=CARTESIAN_POINT('Ctrl Pts',(0.669372269474378,0.101239536626733,
2.53879048903431));
#26478=CARTESIAN_POINT('Ctrl Pts',(0.658418233365987,0.213249763289549,
2.37039231402393));
#26479=CARTESIAN_POINT('Ctrl Pts',(0.647464197257598,0.135184233775625,
2.18381776051518));
#26480=CARTESIAN_POINT('Ctrl Pts',(0.636510161149208,-0.0633748208679874,
2.1453664909722));
#26481=CARTESIAN_POINT('Ctrl Pts',(0.625556125040818,-0.205446266704147,
2.28931055040113));
#26482=CARTESIAN_POINT('Ctrl Pts',(0.614602088932428,-0.164397082111091,
2.48734977756575));
#26483=CARTESIAN_POINT('Ctrl Pts',(0.603648052824038,0.0231831822083779,
2.56296338615472));
#26484=CARTESIAN_POINT('Ctrl Pts',(0.592694016715648,0.190101202472408,
2.44876005223608));
#26485=CARTESIAN_POINT('Ctrl Pts',(0.581739980607259,0.187573349179968,
2.2465221043899));
#26486=CARTESIAN_POINT('Ctrl Pts',(0.570785944498868,0.0178621511754463,
2.13653064821237));
#26487=CARTESIAN_POINT('Ctrl Pts',(0.559831908390479,-0.167782382550835,
2.21678370639397));
#26488=CARTESIAN_POINT('Ctrl Pts',(0.548877872282088,-0.203853376145018,
2.41582942575652));
#26489=CARTESIAN_POINT('Ctrl Pts',(0.537923836173699,-0.0582717589659708,
2.55609455260858));
#26490=CARTESIAN_POINT('Ctrl Pts',(0.526969800065308,0.139343582909784,
2.51287003818356));
#26491=CARTESIAN_POINT('Ctrl Pts',(0.516015763956919,0.212570822922687,
2.32404727633118));
#26492=CARTESIAN_POINT('Ctrl Pts',(0.508713073217992,0.135321818010725,
2.2142903811132));
#26493=CARTESIAN_POINT('Ctrl Pts',(0.505061727848529,0.082032222035417,
2.18740481303031));
#26494=CARTESIAN_POINT('Ctrl Pts',(0.9246,0.175382131162755,2.26384741403295));
#26495=CARTESIAN_POINT('Ctrl Pts',(0.920948654630537,0.147146138548361,
2.20636697389733));
#26496=CARTESIAN_POINT('Ctrl Pts',(0.913645963891609,0.0302731254102407,
2.12223405471588));
#26497=CARTESIAN_POINT('Ctrl Pts',(0.90269192778322,-0.173147373407442,
2.19864027153952));
#26498=CARTESIAN_POINT('Ctrl Pts',(0.89173789167483,-0.221780123875491,
2.41016345103765));
#26499=CARTESIAN_POINT('Ctrl Pts',(0.88078385556644,-0.0729563380969478,
2.56795752352517));
#26500=CARTESIAN_POINT('Ctrl Pts',(0.86982981945805,0.141007563524369,2.53153223318615));
#26501=CARTESIAN_POINT('Ctrl Pts',(0.85887578334966,0.229230625160392,2.33327538882471));
#26502=CARTESIAN_POINT('Ctrl Pts',(0.84792174724127,0.113162513157343,2.14993916039833));
#26503=CARTESIAN_POINT('Ctrl Pts',(0.836967711132881,-0.103785194132055,
2.14491612976786));
#26504=CARTESIAN_POINT('Ctrl Pts',(0.82601367502449,-0.228218764915372,
2.32269376819669));
#26505=CARTESIAN_POINT('Ctrl Pts',(0.815059638916101,-0.149238068465566,
2.52480848786541));
#26506=CARTESIAN_POINT('Ctrl Pts',(0.80410560280771,0.0627647454037258,
2.5711122190708));
#26507=CARTESIAN_POINT('Ctrl Pts',(0.793151566699321,0.218822559259003,
2.42033176164835));
#26508=CARTESIAN_POINT('Ctrl Pts',(0.782197530590931,0.179837962765066,
2.2068627925931));
#26509=CARTESIAN_POINT('Ctrl Pts',(0.771243494482542,-0.0194416757950376,
2.12097605453008));
#26510=CARTESIAN_POINT('Ctrl Pts',(0.760289458374151,-0.201392259367717,
2.23922506423723));
#26511=CARTESIAN_POINT('Ctrl Pts',(0.749335422265762,-0.203836141138318,
2.45621095903406));
#26512=CARTESIAN_POINT('Ctrl Pts',(0.73838138615737,-0.0245949226222939,
2.57852795910941));
#26513=CARTESIAN_POINT('Ctrl Pts',(0.727427350048983,0.176568447645139,
2.49715134904521));
#26514=CARTESIAN_POINT('Ctrl Pts',(0.71647331394059,0.220351245171909,2.284614476127));
#26515=CARTESIAN_POINT('Ctrl Pts',(0.705519277832203,0.0677285780187295,
2.13035761406204));
#26516=CARTESIAN_POINT('Ctrl Pts',(0.69456524172381,-0.145262532199525,
2.17187438991369));
#26517=CARTESIAN_POINT('Ctrl Pts',(0.683611205615423,-0.228776936739271,
2.37215968252717));
#26518=CARTESIAN_POINT('Ctrl Pts',(0.672657169507031,-0.108375810329121,
2.55269342364419));
#26519=CARTESIAN_POINT('Ctrl Pts',(0.661703133398642,0.108623805931346,
2.55256060157758));
#26520=CARTESIAN_POINT('Ctrl Pts',(0.650749097290252,0.228803900870016,
2.3718797007062));
#26521=CARTESIAN_POINT('Ctrl Pts',(0.639795061181862,0.145044381512348,
2.17169666187242));
#26522=CARTESIAN_POINT('Ctrl Pts',(0.628841025073472,-0.0679972911006022,
2.13044081085001));
#26523=CARTESIAN_POINT('Ctrl Pts',(0.617886988965083,-0.220431228227273,
2.28488394736916));
#26524=CARTESIAN_POINT('Ctrl Pts',(0.606932952856692,-0.176387973887657,
2.49736787701848));
#26525=CARTESIAN_POINT('Ctrl Pts',(0.595978916748303,0.0248741308878026,
2.57849663579005));
#26526=CARTESIAN_POINT('Ctrl Pts',(0.585024880639912,0.203966916608997,
2.45596347143917));
#26527=CARTESIAN_POINT('Ctrl Pts',(0.574070844531523,0.201254685255417,
2.23897457233158));
#26528=CARTESIAN_POINT('Ctrl Pts',(0.563116808423133,0.0191649913408013,
2.12096049415593));
#26529=CARTESIAN_POINT('Ctrl Pts',(0.552162772314743,-0.180020193376589,
2.2070670974433));
#26530=CARTESIAN_POINT('Ctrl Pts',(0.541208736206353,-0.218722154472792,
2.42063093141479));
#26531=CARTESIAN_POINT('Ctrl Pts',(0.530254700097963,-0.0625220190461283,
2.5711267991931));
#26532=CARTESIAN_POINT('Ctrl Pts',(0.519300663989573,0.149507107717974,
2.5247495495254));
#26533=CARTESIAN_POINT('Ctrl Pts',(0.508346627881183,0.228075439548419,
2.32215432119582));
#26534=CARTESIAN_POINT('Ctrl Pts',(0.501043937142257,0.145192000947903,
2.20439191252596));
#26535=CARTESIAN_POINT('Ctrl Pts',(0.497392591772793,0.0880155368484699,
2.17554534894914));
#26536=CARTESIAN_POINT('Ctrl Pts',(0.562186969212423,8.98932785041182E-5,
2.15435395233057));
#26537=CARTESIAN_POINT('Ctrl Pts',(0.55884557024653,-0.0583093023980897,
2.15468856527743));
#26538=CARTESIAN_POINT('Ctrl Pts',(0.555504171280636,-0.116990661393897,
2.18260451055754));
#26539=CARTESIAN_POINT('Ctrl Pts',(0.552162772314743,-0.153272989439724,
2.22830996922398));
#26540=CARTESIAN_POINT('Ctrl Pts',(0.54851142694528,-0.192920847075323,
2.27825504210046));
#26541=CARTESIAN_POINT('Ctrl Pts',(0.544860081575816,-0.205821500774057,
2.34944298675763));
#26542=CARTESIAN_POINT('Ctrl Pts',(0.541208736206353,-0.18623847171898,
2.41011960371593));
#26543=CARTESIAN_POINT('Ctrl Pts',(0.53755739083689,-0.166655442663903,
2.47079622067423));
#26544=CARTESIAN_POINT('Ctrl Pts',(0.533906045467426,-0.114588730855015,
2.52096150993366));
#26545=CARTESIAN_POINT('Ctrl Pts',(0.530254700097963,-0.0532171871565546,
2.5383146129521));
#26546=CARTESIAN_POINT('Ctrl Pts',(0.526969800065309,0.00199517034463643,
2.55392617606213));
#26547=CARTESIAN_POINT('Ctrl Pts',(0.523684900032654,0.0647384302451143,
2.54298106678724));
#26548=CARTESIAN_POINT('Ctrl Pts',(0.5204,0.112041393629813,2.51041297594259));
#26549=CARTESIAN_POINT('',(0.9246,-0.126741110252901,2.25945345876159));
#26550=CARTESIAN_POINT('Ctrl Pts',(0.9246,-0.126741110252901,2.25945345876159));
#26551=CARTESIAN_POINT('Ctrl Pts',(0.9246,-0.124304124022258,2.25488172588014));
#26552=CARTESIAN_POINT('Ctrl Pts',(0.9246,-0.121633769967844,2.25045043925615));
#26553=CARTESIAN_POINT('Ctrl Pts',(0.9246,-0.118734751471793,2.2461800207472));
#26554=CARTESIAN_POINT('Ctrl Pts',(0.9246,-0.114974511847176,2.24064097471734));
#26555=CARTESIAN_POINT('Ctrl Pts',(0.9246,-0.110829871551607,2.23537234093936));
#26556=CARTESIAN_POINT('Ctrl Pts',(0.9246,-0.106345035557317,2.23038504832899));
#26557=CARTESIAN_POINT('Ctrl Pts',(0.9246,-0.103023561747274,2.22669145467038));
#26558=CARTESIAN_POINT('Ctrl Pts',(0.9246,-0.099513421358034,2.2231511932741));
#26559=CARTESIAN_POINT('Ctrl Pts',(0.9246,-0.0958481261183665,2.21978442243891));
#26560=CARTESIAN_POINT('Ctrl Pts',(0.9246,-0.0890698117805493,2.21355817611166));
#26561=CARTESIAN_POINT('Ctrl Pts',(0.9246,-0.0817516800897092,2.20791171578257));
#26562=CARTESIAN_POINT('Ctrl Pts',(0.9246,-0.0739985396384171,2.2028752168707));
#26563=CARTESIAN_POINT('Ctrl Pts',(0.9246,-0.0698919378516735,2.20020753716589));
#26564=CARTESIAN_POINT('Ctrl Pts',(0.9246,-0.0656597737776223,2.19771002099059));
#26565=CARTESIAN_POINT('Ctrl Pts',(0.9246,-0.0613394413265084,2.1954000414296));
#26566=CARTESIAN_POINT('Ctrl Pts',(0.9246,-0.0510345828658487,2.18989027737962));
#26567=CARTESIAN_POINT('Ctrl Pts',(0.9246,-0.0402077092576111,2.18542802572008));
#26568=CARTESIAN_POINT('Ctrl Pts',(0.9246,-0.029053385574336,2.1820750264314));
#26569=CARTESIAN_POINT('Ctrl Pts',(0.9246,-0.0239640761508618,2.18054517564338));
#26570=CARTESIAN_POINT('Ctrl Pts',(0.9246,-0.0188060444905203,2.1792467236037));
#26571=CARTESIAN_POINT('Ctrl Pts',(0.9246,-0.0135956684926093,2.17818840646918));
#26572=CARTESIAN_POINT('Ctrl Pts',(0.9246,-0.0090193919946775,2.17725888586799));
#26573=CARTESIAN_POINT('Ctrl Pts',(0.9246,-0.00439842751910679,2.17651455635539));
#26574=CARTESIAN_POINT('Ctrl Pts',(0.9246,0.000228106976056453,2.17596483471338));
#26575=CARTESIAN_POINT('Ctrl Pts',(0.9246,0.00784207747715569,2.17506014798285));
#26576=CARTESIAN_POINT('Ctrl Pts',(0.9246,0.0154840912914549,2.17467851448771));
#26577=CARTESIAN_POINT('Ctrl Pts',(0.9246,0.0231034225456308,2.17483850328635));
#26578=CARTESIAN_POINT('Ctrl Pts',(0.9246,0.0308943277984289,2.1750020947526));
#26579=CARTESIAN_POINT('Ctrl Pts',(0.9246,0.038661730991992,2.17573174383391));
#26580=CARTESIAN_POINT('Ctrl Pts',(0.9246,0.0463653400536272,2.17699151048238));
#26581=CARTESIAN_POINT('Ctrl Pts',(0.9246,0.0507498095388217,2.1777085001926));
#26582=CARTESIAN_POINT('Ctrl Pts',(0.9246,0.0551136501323604,2.17859740678896));
#26583=CARTESIAN_POINT('Ctrl Pts',(0.9246,0.0594494767860557,2.17965309039764));
#26584=CARTESIAN_POINT('Ctrl Pts',(0.9246,0.0631992337756272,2.18056607823284));
#26585=CARTESIAN_POINT('Ctrl Pts',(0.9246,0.0669204105008384,2.1816021115383));
#26586=CARTESIAN_POINT('Ctrl Pts',(0.9246,0.0706019654180724,2.18275450707801));
#26587=CARTESIAN_POINT('Ctrl Pts',(0.9246,0.0813244048177332,2.18611083113583));
#26588=CARTESIAN_POINT('Ctrl Pts',(0.9246,0.0917275081526179,2.19045541621774));
#26589=CARTESIAN_POINT('Ctrl Pts',(0.9246,0.101696782898373,2.19568714303042));
#26590=CARTESIAN_POINT('Ctrl Pts',(0.9246,0.109000366691416,2.19951995495838));
#26591=CARTESIAN_POINT('Ctrl Pts',(0.9246,0.116071340784156,2.20382979183443));
#26592=CARTESIAN_POINT('Ctrl Pts',(0.9246,0.122862456295835,2.2085889147266));
#26593=CARTESIAN_POINT('Ctrl Pts',(0.9246,0.125551050441307,2.21047304553302));
#26594=CARTESIAN_POINT('Ctrl Pts',(0.9246,0.128194234915945,2.21242684283041));
#26595=CARTESIAN_POINT('Ctrl Pts',(0.9246,0.13078174991918,2.21444248700447));
#26596=CARTESIAN_POINT('Ctrl Pts',(0.9246,0.140899810628574,2.22232433893425));
#26597=CARTESIAN_POINT('Ctrl Pts',(0.9246,0.150200729496614,2.23117056966092));
#26598=CARTESIAN_POINT('Ctrl Pts',(0.9246,0.158522385857352,2.2408616404524));
#26599=CARTESIAN_POINT('Ctrl Pts',(0.9246,0.164709234946706,2.24806659940553));
#26600=CARTESIAN_POINT('Ctrl Pts',(0.9246,0.170354866494887,2.25573972458116));
#26601=CARTESIAN_POINT('Ctrl Pts',(0.9246,0.175382131162755,2.26384741403295));
#26602=CARTESIAN_POINT('Ctrl Pts',(0.9246,-0.1267411102529,2.25945345876159));
#26603=CARTESIAN_POINT('Ctrl Pts',(0.921315099967346,-0.153066813359842,
2.29683117428655));
#26604=CARTESIAN_POINT('Ctrl Pts',(0.914378854565228,-0.172586882197048,
2.4020958249901));
#26605=CARTESIAN_POINT('Ctrl Pts',(0.903791263793647,-0.0580775762076774,
2.52350712786254));
#26606=CARTESIAN_POINT('Ctrl Pts',(0.892837227685257,0.112250391536416,
2.49451043435059));
#26607=CARTESIAN_POINT('Ctrl Pts',(0.881883191576867,0.182481185996413,
2.33668621664117));
#26608=CARTESIAN_POINT('Ctrl Pts',(0.872668908161658,0.104758862680348,
2.2139193569465));
#26609=CARTESIAN_POINT('Ctrl Pts',(0.867105970115912,0.0267685152039638,
2.19471498811069));
#26610=CARTESIAN_POINT('Ctrl Pts',(0.865194377439629,-1.79285551041419E-5,
2.19468551470809));
#26611=CARTESIAN_POINT('Origin',(0.9246,2.59090492670967E-17,2.35));
#26612=CARTESIAN_POINT('',(0.9246,-2.39295984553393E-17,2.1546));
#26613=CARTESIAN_POINT('Origin',(0.9246,0.,2.35));
#26614=CARTESIAN_POINT('Origin',(0.9246,0.,2.35));
#26615=CARTESIAN_POINT('',(0.9246,-0.126612599672286,2.44036067786502));
#26616=CARTESIAN_POINT('Ctrl Pts',(0.9246,0.175579315085692,2.4363567917616));
#26617=CARTESIAN_POINT('Ctrl Pts',(0.9246,0.172231987765182,2.44182477166145));
#26618=CARTESIAN_POINT('Ctrl Pts',(0.9246,0.168608550730546,2.44710587712298));
#26619=CARTESIAN_POINT('Ctrl Pts',(0.9246,0.164708478737988,2.45217506292884));
#26620=CARTESIAN_POINT('Ctrl Pts',(0.9246,0.158764977139952,2.45990023159121));
#26621=CARTESIAN_POINT('Ctrl Pts',(0.9246,0.152179218509756,2.46713401293529));
#26622=CARTESIAN_POINT('Ctrl Pts',(0.9246,0.145034638687745,2.47383351561557));
#26623=CARTESIAN_POINT('Ctrl Pts',(0.9246,0.142072703988846,2.47661093429496));
#26624=CARTESIAN_POINT('Ctrl Pts',(0.9246,0.139016477261661,2.47929437243742));
#26625=CARTESIAN_POINT('Ctrl Pts',(0.9246,0.135878681353299,2.48187551125661));
#26626=CARTESIAN_POINT('Ctrl Pts',(0.9246,0.130129041557607,2.48660514278983));
#26627=CARTESIAN_POINT('Ctrl Pts',(0.9246,0.124099585925552,2.49099741573807));
#26628=CARTESIAN_POINT('Ctrl Pts',(0.9246,0.117828170685741,2.49503327073206));
#26629=CARTESIAN_POINT('Ctrl Pts',(0.9246,0.113097205680066,2.49807779704939));
#26630=CARTESIAN_POINT('Ctrl Pts',(0.9246,0.108228470452361,2.50091938744955));
#26631=CARTESIAN_POINT('Ctrl Pts',(0.9246,0.103237746210791,2.50354755952374));
#26632=CARTESIAN_POINT('Ctrl Pts',(0.9246,0.0995081913357007,2.50551158548419));
#26633=CARTESIAN_POINT('Ctrl Pts',(0.9246,0.095718014229134,2.50735230916665));
#26634=CARTESIAN_POINT('Ctrl Pts',(0.9246,0.0918791218561784,2.50906440216875));
#26635=CARTESIAN_POINT('Ctrl Pts',(0.9246,0.0807315995386604,2.51403604322986));
#26636=CARTESIAN_POINT('Ctrl Pts',(0.9246,0.0691604417837671,2.51793368204044));
#26637=CARTESIAN_POINT('Ctrl Pts',(0.9246,0.0573325104935312,2.52065673448287));
#26638=CARTESIAN_POINT('Ctrl Pts',(0.9246,0.0517514512541242,2.52194161825673));
#26639=CARTESIAN_POINT('Ctrl Pts',(0.9246,0.0461131794767607,2.52296425202055));
#26640=CARTESIAN_POINT('Ctrl Pts',(0.9246,0.0404358087089947,2.52370990579393));
#26641=CARTESIAN_POINT('Ctrl Pts',(0.9246,0.0362131138627409,2.52426450553292));
#26642=CARTESIAN_POINT('Ctrl Pts',(0.9246,0.0319671072283097,2.52466551133679));
#26643=CARTESIAN_POINT('Ctrl Pts',(0.9246,0.0277269183658541,2.52490584661354));
#26644=CARTESIAN_POINT('Ctrl Pts',(0.9246,0.0203386643257472,2.52532461524319));
#26645=CARTESIAN_POINT('Ctrl Pts',(0.9246,0.0129531623571097,2.52525855005896));
#26646=CARTESIAN_POINT('Ctrl Pts',(0.9246,0.00560966548235301,2.52468156733611));
#26647=CARTESIAN_POINT('Ctrl Pts',(0.9246,-0.00111838109498682,2.5241529408929));
#26648=CARTESIAN_POINT('Ctrl Pts',(0.9246,-0.00781125354088175,2.52319524983962));
#26649=CARTESIAN_POINT('Ctrl Pts',(0.9246,-0.0144367695388186,2.52182652343633));
#26650=CARTESIAN_POINT('Ctrl Pts',(0.9246,-0.0194845103225483,2.52078374033993));
#26651=CARTESIAN_POINT('Ctrl Pts',(0.9246,-0.0244931239656314,2.51950225818089));
#26652=CARTESIAN_POINT('Ctrl Pts',(0.9246,-0.0294470198886176,2.51798836500374));
#26653=CARTESIAN_POINT('Ctrl Pts',(0.9246,-0.0327263379688084,2.51698621692787));
#26654=CARTESIAN_POINT('Ctrl Pts',(0.9246,-0.0359767748311459,2.51588354002561));
#26655=CARTESIAN_POINT('Ctrl Pts',(0.9246,-0.0391872039422838,2.5146856379879));
#26656=CARTESIAN_POINT('Ctrl Pts',(0.9246,-0.0483434462127441,2.51126918464356));
#26657=CARTESIAN_POINT('Ctrl Pts',(0.9246,-0.0571935346348361,2.50707428148216));
#26658=CARTESIAN_POINT('Ctrl Pts',(0.9246,-0.0656377525465968,2.50215785253157));
#26659=CARTESIAN_POINT('Ctrl Pts',(0.9246,-0.0707606060416182,2.49917520268812));
#26660=CARTESIAN_POINT('Ctrl Pts',(0.9246,-0.0757337923895695,2.49592655376489));
#26661=CARTESIAN_POINT('Ctrl Pts',(0.9246,-0.0805312179131897,2.4924215291976));
#26662=CARTESIAN_POINT('Ctrl Pts',(0.9246,-0.0832471843025241,2.49043722972872));
#26663=CARTESIAN_POINT('Ctrl Pts',(0.9246,-0.0859085907169423,2.48836919294223));
#26664=CARTESIAN_POINT('Ctrl Pts',(0.9246,-0.0885041357554648,2.4862239808703));
#26665=CARTESIAN_POINT('Ctrl Pts',(0.9246,-0.0968642111344724,2.4793143975808));
#26666=CARTESIAN_POINT('Ctrl Pts',(0.9246,-0.104507209259633,2.47163878643969));
#26667=CARTESIAN_POINT('Ctrl Pts',(0.9246,-0.111283835708874,2.46326800079988));
#26668=CARTESIAN_POINT('Ctrl Pts',(0.9246,-0.117064352600238,2.45612765329108));
#26669=CARTESIAN_POINT('Ctrl Pts',(0.9246,-0.122214313018595,2.44848056071584));
#26670=CARTESIAN_POINT('Ctrl Pts',(0.9246,-0.126612599672285,2.44036067786502));
#26671=CARTESIAN_POINT('Origin',(0.9246,0.,2.35));
#26672=CARTESIAN_POINT('Origin',(1.05400562256037,0.,2.35));
#26673=CARTESIAN_POINT('Ctrl Pts',(0.9246,-0.126612599672285,2.44036067786502));
#26674=CARTESIAN_POINT('Ctrl Pts',(0.920948654630537,-0.096997430212323,
2.48185719696664));
#26675=CARTESIAN_POINT('Ctrl Pts',(0.91364596389161,0.00568860837306084,
2.53282102514772));
#26676=CARTESIAN_POINT('Ctrl Pts',(0.90269192778322,0.155584940979638,2.44648887334014));
#26677=CARTESIAN_POINT('Ctrl Pts',(0.89173789167483,0.166419612567735,2.27405040496673));
#26678=CARTESIAN_POINT('Ctrl Pts',(0.883842456600547,0.0674478883148535,
2.19859243881242));
#26679=CARTESIAN_POINT('Ctrl Pts',(0.879598366895727,0.00838374554634853,
2.19427942878313));
#26680=CARTESIAN_POINT('Ctrl Pts',(0.87900562256037,0.000124190176919186,
2.19434837072514));
#26681=CARTESIAN_POINT('Ctrl Pts',(0.947607408227207,-0.159049193030952,
2.46350997399437));
#26682=CARTESIAN_POINT('Ctrl Pts',(0.943956062857743,-0.121846980800308,
2.51563739175366));
#26683=CARTESIAN_POINT('Ctrl Pts',(0.936653372118817,0.00714595998775946,
2.57965752692937));
#26684=CARTESIAN_POINT('Ctrl Pts',(0.925699336010427,0.19544389242958,2.47120813790205));
#26685=CARTESIAN_POINT('Ctrl Pts',(0.914745299902037,0.209054273839508,
2.25459305130504));
#26686=CARTESIAN_POINT('Ctrl Pts',(0.903791263793647,0.036564329522591,
2.12308336529646));
#26687=CARTESIAN_POINT('Ctrl Pts',(0.892837227685257,-0.168635162060087,
2.19379733502253));
#26688=CARTESIAN_POINT('Ctrl Pts',(0.881883191576868,-0.22346517637455,
2.40375636415297));
#26689=CARTESIAN_POINT('Ctrl Pts',(0.870929155468477,-0.0791446139402059,
2.5657921277133));
#26690=CARTESIAN_POINT('Ctrl Pts',(0.859975119360087,0.135735248705182,
2.53549049134978));
#26691=CARTESIAN_POINT('Ctrl Pts',(0.849021083251697,0.229622539590993,
2.33985357530928));
#26692=CARTESIAN_POINT('Ctrl Pts',(0.838067047143308,0.11884455109742,2.15326158747437));
#26693=CARTESIAN_POINT('Ctrl Pts',(0.827113011034917,-0.0978650376008603,
2.14202768607467));
#26694=CARTESIAN_POINT('Ctrl Pts',(0.816158974926528,-0.227343663615742,
2.31616583232657));
#26695=CARTESIAN_POINT('Ctrl Pts',(0.805204938818137,-0.154184798574543,
2.52046120780869));
#26696=CARTESIAN_POINT('Ctrl Pts',(0.794250902709748,0.0564037123155049,
2.57281963603689));
#26697=CARTESIAN_POINT('Ctrl Pts',(0.783296866601358,0.216717825635759,
2.42657241872938));
#26698=CARTESIAN_POINT('Ctrl Pts',(0.772342830492967,0.183865118597134,
2.21207400158005));
#26699=CARTESIAN_POINT('Ctrl Pts',(0.761388794384579,-0.0128719385109397,
2.12051301962112));
#26700=CARTESIAN_POINT('Ctrl Pts',(0.750434758276188,-0.19813584580039,
2.23350044847083));
#26701=CARTESIAN_POINT('Ctrl Pts',(0.739480722167799,-0.206795533067443,
2.45032730502815));
#26702=CARTESIAN_POINT('Ctrl Pts',(0.728526686059409,-0.031132354710069,
2.57772952623906));
#26703=CARTESIAN_POINT('Ctrl Pts',(0.717572649951018,0.172279990092259,
2.50214980746404));
#26704=CARTESIAN_POINT('Ctrl Pts',(0.706618613842629,0.222134186250392,
2.29095455764139));
#26705=CARTESIAN_POINT('Ctrl Pts',(0.695664577734239,0.0739937252264801,
2.13238820917977));
#26706=CARTESIAN_POINT('Ctrl Pts',(0.684710541625849,-0.140099470470165,
2.16778559433366));
#26707=CARTESIAN_POINT('Ctrl Pts',(0.673756505517459,-0.229317981351449,
2.36559590957524));
#26708=CARTESIAN_POINT('Ctrl Pts',(0.662802469409069,-0.114138643817405,
2.54950525172684));
#26709=CARTESIAN_POINT('Ctrl Pts',(0.651848433300679,0.102775627973098,
2.55558954881783));
#26710=CARTESIAN_POINT('Ctrl Pts',(0.640894397192289,0.228083298654142,
2.37842635782365));
#26711=CARTESIAN_POINT('Ctrl Pts',(0.629940361083899,0.150093116511318,
2.17592505446052));
#26712=CARTESIAN_POINT('Ctrl Pts',(0.618986324975509,-0.0616782521441111,
2.12858352853803));
#26713=CARTESIAN_POINT('Ctrl Pts',(0.60803228886712,-0.218476302610795,
2.27859352046379));
#26714=CARTESIAN_POINT('Ctrl Pts',(0.597078252758729,-0.180535547996485,
2.49225690917627));
#26715=CARTESIAN_POINT('Ctrl Pts',(0.58612421665034,0.0183128246430198,
2.57910930184663));
#26716=CARTESIAN_POINT('Ctrl Pts',(0.57517018054195,0.200856123874476,2.46177615099481));
#26717=CARTESIAN_POINT('Ctrl Pts',(0.564216144433559,0.204335629037752,
2.24476188901181));
#26718=CARTESIAN_POINT('Ctrl Pts',(0.553262108325171,0.0257537850119573,
2.12165176193497));
#26719=CARTESIAN_POINT('Ctrl Pts',(0.542308072216779,-0.17591953461002,
2.20187152493763));
#26720=CARTESIAN_POINT('Ctrl Pts',(0.53135403610839,-0.220517757106366,
2.41454117461156));
#26721=CARTESIAN_POINT('Ctrl Pts',(0.524051345369463,-0.119597839472195,
2.51726861352534));
#26722=CARTESIAN_POINT('Ctrl Pts',(0.5204,-0.0584934195161147,2.53643948045763));
#26723=CARTESIAN_POINT('Ctrl Pts',(0.939938272151471,-0.14823699524473,
2.45579354195125));
#26724=CARTESIAN_POINT('Ctrl Pts',(0.936286926782008,-0.11356379727098,
2.50437732682465));
#26725=CARTESIAN_POINT('Ctrl Pts',(0.928984236043081,0.00666017611619341,
2.56404535966882));
#26726=CARTESIAN_POINT('Ctrl Pts',(0.918030199934691,0.182157575279599,
2.46296838304809));
#26727=CARTESIAN_POINT('Ctrl Pts',(0.907076163826302,0.19484272008225,2.26107883585894));
#26728=CARTESIAN_POINT('Ctrl Pts',(0.896122127717911,0.0340786786671227,
2.13850920612372));
#26729=CARTESIAN_POINT('Ctrl Pts',(0.885168091609522,-0.157171308071526,
2.20441602522955));
#26730=CARTESIAN_POINT('Ctrl Pts',(0.874214055501132,-0.208273966414595,
2.40010199514667));
#26731=CARTESIAN_POINT('Ctrl Pts',(0.863260019392742,-0.0737643463429399,
2.55112253322443));
#26732=CARTESIAN_POINT('Ctrl Pts',(0.852305983284351,0.126507937785869,
2.52288080851067));
#26733=CARTESIAN_POINT('Ctrl Pts',(0.841351947175962,0.214012750777105,
2.34054333140604));
#26734=CARTESIAN_POINT('Ctrl Pts',(0.830397911067572,0.110765473374403,
2.16663590637431));
#26735=CARTESIAN_POINT('Ctrl Pts',(0.819443874959182,-0.0912121516431767,
2.1561656879681));
#26736=CARTESIAN_POINT('Ctrl Pts',(0.808489838850792,-0.211888793272707,
2.31846588620202));
#26737=CARTESIAN_POINT('Ctrl Pts',(0.797535802742403,-0.143703283352442,
2.50887321884387));
#26738=CARTESIAN_POINT('Ctrl Pts',(0.786581766634012,0.0525693760211127,
2.55767231004564));
#26739=CARTESIAN_POINT('Ctrl Pts',(0.775627730525623,0.201985302006306,
2.42136700950665));
#26740=CARTESIAN_POINT('Ctrl Pts',(0.764673694417233,0.171365928941563,
2.22145024012839));
#26741=CARTESIAN_POINT('Ctrl Pts',(0.753719658308842,-0.0119969014081408,
2.13611359309109));
#26742=CARTESIAN_POINT('Ctrl Pts',(0.742765622200453,-0.184666529090828,
2.24142011262716));
#26743=CARTESIAN_POINT('Ctrl Pts',(0.731811586092063,-0.192737528985666,
2.44350703360992));
#26744=CARTESIAN_POINT('Ctrl Pts',(0.720857549983673,-0.0290159706513922,
2.56224842487327));
#26745=CARTESIAN_POINT('Ctrl Pts',(0.709903513875283,0.160568359923073,
2.4918066313681));
#26746=CARTESIAN_POINT('Ctrl Pts',(0.698949477766892,0.207033457280624,
2.29496847930292));
#26747=CARTESIAN_POINT('Ctrl Pts',(0.687995441658504,0.0689636161335506,
2.14718150475157));
#26748=CARTESIAN_POINT('Ctrl Pts',(0.677041405550113,-0.130575478832096,
2.18017256817501));
#26749=CARTESIAN_POINT('Ctrl Pts',(0.666087369441724,-0.213728896471109,
2.36453569634329));
#26750=CARTESIAN_POINT('Ctrl Pts',(0.655133333333333,-0.106379474666734,
2.53594284251273));
#26751=CARTESIAN_POINT('Ctrl Pts',(0.644179297224944,0.0957889190431628,
2.54161352780044));
#26752=CARTESIAN_POINT('Ctrl Pts',(0.633225261116553,0.21257814776474,2.37649392800571));
#26753=CARTESIAN_POINT('Ctrl Pts',(0.622271225008164,0.139889754701397,
2.1877587060807));
#26754=CARTESIAN_POINT('Ctrl Pts',(0.611317188899773,-0.0574853515164367,
2.14363546710466));
#26755=CARTESIAN_POINT('Ctrl Pts',(0.600363152791384,-0.203624237344606,
2.28344774804741));
#26756=CARTESIAN_POINT('Ctrl Pts',(0.589409116682994,-0.168262703254657,
2.48258625439859));
#26757=CARTESIAN_POINT('Ctrl Pts',(0.578455080574604,0.0170679149500409,
2.56353440304317));
#26758=CARTESIAN_POINT('Ctrl Pts',(0.567501044466214,0.187201882086012,
2.45417758460596));
#26759=CARTESIAN_POINT('Ctrl Pts',(0.556547008357824,0.190444849752262,
2.251915998058));
#26760=CARTESIAN_POINT('Ctrl Pts',(0.545592972249434,0.0240030372590971,
2.13717492346157));
#26761=CARTESIAN_POINT('Ctrl Pts',(0.534638936141044,-0.163960487434638,
2.21194133000627));
#26762=CARTESIAN_POINT('Ctrl Pts',(0.523684900032654,-0.205526913331735,
2.41015365190895));
#26763=CARTESIAN_POINT('Ctrl Pts',(0.516382209293728,-0.111467553046117,
2.50589765779524));
#26764=CARTESIAN_POINT('Ctrl Pts',(0.512730863924264,-0.0545170244841849,
2.52376528513823));
#26765=CARTESIAN_POINT('Ctrl Pts',(0.932269136075736,-0.137424797458508,
2.44807710990814));
#26766=CARTESIAN_POINT('Ctrl Pts',(0.928617790706272,-0.105280613741651,
2.49311726189564));
#26767=CARTESIAN_POINT('Ctrl Pts',(0.921315099967346,0.00617439224462701,
2.54843319240827));
#26768=CARTESIAN_POINT('Ctrl Pts',(0.910361063858956,0.168871258129619,
2.45472862819411));
#26769=CARTESIAN_POINT('Ctrl Pts',(0.899407027750566,0.180631166324993,
2.26756462041284));
#26770=CARTESIAN_POINT('Ctrl Pts',(0.888452991642176,0.0315930278116549,
2.15393504695097));
#26771=CARTESIAN_POINT('Ctrl Pts',(0.877498955533787,-0.145707454082965,
2.21503471543656));
#26772=CARTESIAN_POINT('Ctrl Pts',(0.866544919425395,-0.19308275645464,
2.39644762614036));
#26773=CARTESIAN_POINT('Ctrl Pts',(0.855590883317007,-0.068384078745674,
2.53645293873556));
#26774=CARTESIAN_POINT('Ctrl Pts',(0.844636847208615,0.117280626866556,
2.51027112567155));
#26775=CARTESIAN_POINT('Ctrl Pts',(0.833682811100227,0.198402961963217,
2.34123308750281));
#26776=CARTESIAN_POINT('Ctrl Pts',(0.822728774991836,0.102686395651387,
2.18001022527425));
#26777=CARTESIAN_POINT('Ctrl Pts',(0.811774738883446,-0.0845592656854929,
2.17030368986152));
#26778=CARTESIAN_POINT('Ctrl Pts',(0.800820702775057,-0.196433922929672,
2.32076594007746));
#26779=CARTESIAN_POINT('Ctrl Pts',(0.789866666666667,-0.133221768130341,
2.49728522987905));
#26780=CARTESIAN_POINT('Ctrl Pts',(0.778912630558277,0.0487350397267202,
2.54252498405439));
#26781=CARTESIAN_POINT('Ctrl Pts',(0.767958594449887,0.187252778376854,
2.41616160028392));
#26782=CARTESIAN_POINT('Ctrl Pts',(0.757004558341496,0.158866739285992,
2.23082647867672));
#26783=CARTESIAN_POINT('Ctrl Pts',(0.746050522233108,-0.0111218643053415,
2.15171416656106));
#26784=CARTESIAN_POINT('Ctrl Pts',(0.735096486124717,-0.171197212381266,
2.24933977678348));
#26785=CARTESIAN_POINT('Ctrl Pts',(0.724142450016327,-0.178679524903889,
2.43668676219168));
#26786=CARTESIAN_POINT('Ctrl Pts',(0.713188413907937,-0.0268995865927155,
2.54676732350748));
#26787=CARTESIAN_POINT('Ctrl Pts',(0.702234377799547,0.148856729753888,
2.48146345527215));
#26788=CARTESIAN_POINT('Ctrl Pts',(0.691280341691157,0.191932728310855,
2.29898240096446));
#26789=CARTESIAN_POINT('Ctrl Pts',(0.680326305582768,0.0639335070406211,
2.16197480032336));
#26790=CARTESIAN_POINT('Ctrl Pts',(0.669372269474378,-0.121051487194027,
2.19255954201638));
#26791=CARTESIAN_POINT('Ctrl Pts',(0.658418233365988,-0.198139811590769,
2.36347548311133));
#26792=CARTESIAN_POINT('Ctrl Pts',(0.647464197257598,-0.0986203055160625,
2.52238043329861));
#26793=CARTESIAN_POINT('Ctrl Pts',(0.636510161149208,0.0888022101132281,
2.52763750678306));
#26794=CARTESIAN_POINT('Ctrl Pts',(0.625556125040818,0.197072996875337,
2.37456149818778));
#26795=CARTESIAN_POINT('Ctrl Pts',(0.614602088932428,0.129686392891475,
2.19959235770088));
#26796=CARTESIAN_POINT('Ctrl Pts',(0.603648052824039,-0.0532924508887624,
2.15868740567129));
#26797=CARTESIAN_POINT('Ctrl Pts',(0.592694016715648,-0.188772172078417,
2.28830197563102));
#26798=CARTESIAN_POINT('Ctrl Pts',(0.581739980607258,-0.155989858512828,
2.47291559962092));
#26799=CARTESIAN_POINT('Ctrl Pts',(0.570785944498869,0.0158230052570621,
2.54795950423971));
#26800=CARTESIAN_POINT('Ctrl Pts',(0.559831908390478,0.173547640297548,
2.44657901821711));
#26801=CARTESIAN_POINT('Ctrl Pts',(0.548877872282089,0.176554070466772,
2.2590701071042));
#26802=CARTESIAN_POINT('Ctrl Pts',(0.537923836173699,0.022252289506237,
2.15269808498817));
#26803=CARTESIAN_POINT('Ctrl Pts',(0.526969800065309,-0.152001440259255,
2.22201113507491));
#26804=CARTESIAN_POINT('Ctrl Pts',(0.516015763956919,-0.190536069557104,
2.40576612920634));
#26805=CARTESIAN_POINT('Ctrl Pts',(0.508713073217992,-0.103337266620039,
2.49452670206514));
#26806=CARTESIAN_POINT('Ctrl Pts',(0.505061727848529,-0.0505406294522551,
2.51109108981882));
#26807=CARTESIAN_POINT('Ctrl Pts',(0.9246,-0.126612599672285,2.44036067786502));
#26808=CARTESIAN_POINT('Ctrl Pts',(0.920948654630537,-0.096997430212323,
2.48185719696664));
#26809=CARTESIAN_POINT('Ctrl Pts',(0.91364596389161,0.00568860837306084,
2.53282102514772));
#26810=CARTESIAN_POINT('Ctrl Pts',(0.90269192778322,0.155584940979638,2.44648887334014));
#26811=CARTESIAN_POINT('Ctrl Pts',(0.89173789167483,0.166419612567735,2.27405040496673));
#26812=CARTESIAN_POINT('Ctrl Pts',(0.880783855566441,0.0291073769561869,
2.16936088777822));
#26813=CARTESIAN_POINT('Ctrl Pts',(0.86982981945805,-0.134243600094404,
2.22565340564358));
#26814=CARTESIAN_POINT('Ctrl Pts',(0.858875783349661,-0.177891546494684,
2.39279325713406));
#26815=CARTESIAN_POINT('Ctrl Pts',(0.847921747241271,-0.0630038111484079,
2.52178334424669));
#26816=CARTESIAN_POINT('Ctrl Pts',(0.83696771113288,0.108053315947243,2.49766144283244));
#26817=CARTESIAN_POINT('Ctrl Pts',(0.826013675024491,0.18279317314933,2.34192284359958));
#26818=CARTESIAN_POINT('Ctrl Pts',(0.815059638916101,0.0946073179283704,
2.1933845441742));
#26819=CARTESIAN_POINT('Ctrl Pts',(0.804105602807711,-0.0779063797278091,
2.18444169175494));
#26820=CARTESIAN_POINT('Ctrl Pts',(0.793151566699321,-0.180979052586637,
2.32306599395291));
#26821=CARTESIAN_POINT('Ctrl Pts',(0.782197530590931,-0.12274025290824,
2.48569724091423));
#26822=CARTESIAN_POINT('Ctrl Pts',(0.771243494482541,0.0449007034323279,
2.52737765806314));
#26823=CARTESIAN_POINT('Ctrl Pts',(0.760289458374152,0.172520254747402,
2.41095619106118));
#26824=CARTESIAN_POINT('Ctrl Pts',(0.749335422265761,0.146367549630421,
2.24020271722506));
#26825=CARTESIAN_POINT('Ctrl Pts',(0.738381386157372,-0.0102468272025424,
2.16731474003104));
#26826=CARTESIAN_POINT('Ctrl Pts',(0.727427350048981,-0.157727895671703,
2.2572594409398));
#26827=CARTESIAN_POINT('Ctrl Pts',(0.716473313940592,-0.164621520822112,
2.42986649077344));
#26828=CARTESIAN_POINT('Ctrl Pts',(0.705519277832201,-0.0247832025340387,
2.53128622214169));
#26829=CARTESIAN_POINT('Ctrl Pts',(0.694565241723812,0.137145099584703,
2.47112027917621));
#26830=CARTESIAN_POINT('Ctrl Pts',(0.683611205615422,0.176831999341087,
2.30299632262599));
#26831=CARTESIAN_POINT('Ctrl Pts',(0.672657169507032,0.0589033979476915,
2.17676809589516));
#26832=CARTESIAN_POINT('Ctrl Pts',(0.661703133398642,-0.111527495555958,
2.20494651585773));
#26833=CARTESIAN_POINT('Ctrl Pts',(0.650749097290252,-0.182550726710429,
2.36241526987937));
#26834=CARTESIAN_POINT('Ctrl Pts',(0.639795061181862,-0.0908611363653908,
2.5088180240845));
#26835=CARTESIAN_POINT('Ctrl Pts',(0.628841025073472,0.0818155011832931,
2.51366148576568));
#26836=CARTESIAN_POINT('Ctrl Pts',(0.617886988965083,0.181567845985935,
2.37262906836985));
#26837=CARTESIAN_POINT('Ctrl Pts',(0.606932952856693,0.119483031081553,
2.21142600932105));
#26838=CARTESIAN_POINT('Ctrl Pts',(0.595978916748302,-0.049099550261088,
2.17373934423792));
#26839=CARTESIAN_POINT('Ctrl Pts',(0.585024880639913,-0.173920106812228,
2.29315620321465));
#26840=CARTESIAN_POINT('Ctrl Pts',(0.574070844531523,-0.143717013770999,
2.46324494484324));
#26841=CARTESIAN_POINT('Ctrl Pts',(0.563116808423133,0.014578095564083,
2.53238460543625));
#26842=CARTESIAN_POINT('Ctrl Pts',(0.552162772314743,0.159893398509083,
2.43898045182826));
#26843=CARTESIAN_POINT('Ctrl Pts',(0.541208736206353,0.162663291181281,
2.2662242161504));
#26844=CARTESIAN_POINT('Ctrl Pts',(0.530254700097963,0.020501541753377,
2.16822124651476));
#26845=CARTESIAN_POINT('Ctrl Pts',(0.519300663989573,-0.140042393083873,
2.23208094014354));
#26846=CARTESIAN_POINT('Ctrl Pts',(0.508346627881183,-0.175545225782473,
2.40137860650373));
#26847=CARTESIAN_POINT('Ctrl Pts',(0.501043937142257,-0.0952069801939604,
2.48315574633504));
#26848=CARTESIAN_POINT('Ctrl Pts',(0.497392591772793,-0.0465642344203253,
2.49841689449941));
#26849=CARTESIAN_POINT('Ctrl Pts',(0.5204,-0.0584934195161159,2.53643948045763));
#26850=CARTESIAN_POINT('Ctrl Pts',(0.524051345369463,-0.119597839472196,
2.51726861352533));
#26851=CARTESIAN_POINT('Ctrl Pts',(0.527702690738927,-0.170057798289281,
2.46590489406845));
#26852=CARTESIAN_POINT('Ctrl Pts',(0.53135403610839,-0.187854740615099,
2.40477809272768));
#26853=CARTESIAN_POINT('Ctrl Pts',(0.535005381477853,-0.205651682940918,
2.34365129138692));
#26854=CARTESIAN_POINT('Ctrl Pts',(0.538656726847316,-0.190785608775469,
2.27276140816228));
#26855=CARTESIAN_POINT('Ctrl Pts',(0.54230807221678,-0.149740351755748,
2.22394650604951));
#26856=CARTESIAN_POINT('Ctrl Pts',(0.545543058407045,-0.113375443427666,
2.18069791731435));
#26857=CARTESIAN_POINT('Ctrl Pts',(0.548778044597311,-0.056461325508588,
2.15477696695928));
#26858=CARTESIAN_POINT('Ctrl Pts',(0.552013030787577,0.000119548669269599,
2.15439909884273));
#26859=CARTESIAN_POINT('Origin',(0.95,0.0577350269189626,2.45));
#26860=CARTESIAN_POINT('',(0.95,0.0577350269189626,2.45));
#26861=CARTESIAN_POINT('',(0.95,0.115470053837925,2.35));
#26862=CARTESIAN_POINT('',(0.95,0.0353627039878646,2.48875));
#26863=CARTESIAN_POINT('',(0.75,0.0577350269189626,2.45));
#26864=CARTESIAN_POINT('',(0.95,0.0577350269189626,2.45));
#26865=CARTESIAN_POINT('',(0.75,0.115470053837925,2.35));
#26866=CARTESIAN_POINT('',(0.75,0.115470053837925,2.35));
#26867=CARTESIAN_POINT('',(0.95,0.115470053837925,2.35));
#26868=CARTESIAN_POINT('Origin',(0.95,-0.0577350269189626,2.45));
#26869=CARTESIAN_POINT('',(0.95,-0.0577350269189626,2.45));
#26870=CARTESIAN_POINT('',(0.95,-0.0288675134594813,2.45));
#26871=CARTESIAN_POINT('',(0.75,-0.0577350269189626,2.45));
#26872=CARTESIAN_POINT('',(0.95,-0.0577350269189626,2.45));
#26873=CARTESIAN_POINT('',(0.75,0.0577350269189626,2.45));
#26874=CARTESIAN_POINT('Origin',(0.95,-0.115470053837925,2.35));
#26875=CARTESIAN_POINT('',(0.95,-0.115470053837925,2.35));
#26876=CARTESIAN_POINT('',(0.95,-0.0642302174473459,2.43875));
#26877=CARTESIAN_POINT('',(0.75,-0.115470053837925,2.35));
#26878=CARTESIAN_POINT('',(0.95,-0.115470053837925,2.35));
#26879=CARTESIAN_POINT('',(0.75,-0.0577350269189626,2.45));
#26880=CARTESIAN_POINT('Origin',(0.95,-0.0577350269189626,2.25));
#26881=CARTESIAN_POINT('',(0.95,-0.0577350269189626,2.25));
#26882=CARTESIAN_POINT('',(0.95,-0.108974863309542,2.33875));
#26883=CARTESIAN_POINT('',(0.75,-0.0577350269189626,2.25));
#26884=CARTESIAN_POINT('',(0.95,-0.0577350269189626,2.25));
#26885=CARTESIAN_POINT('',(0.75,-0.115470053837925,2.35));
#26886=CARTESIAN_POINT('Origin',(0.95,0.0577350269189626,2.25));
#26887=CARTESIAN_POINT('',(0.95,0.0577350269189626,2.25));
#26888=CARTESIAN_POINT('',(0.95,0.0288675134594813,2.25));
#26889=CARTESIAN_POINT('',(0.75,0.0577350269189626,2.25));
#26890=CARTESIAN_POINT('',(0.95,0.0577350269189626,2.25));
#26891=CARTESIAN_POINT('',(0.75,-0.0577350269189626,2.25));
#26892=CARTESIAN_POINT('Origin',(0.95,0.115470053837925,2.35));
#26893=CARTESIAN_POINT('',(0.95,0.137842376769023,2.38875));
#26894=CARTESIAN_POINT('',(0.75,0.0577350269189626,2.25));
#26895=CARTESIAN_POINT('Origin',(0.75,0.,2.35));
#26896=CARTESIAN_POINT('Origin',(0.95,0.,2.52));
#26897=CARTESIAN_POINT('',(0.95,-2.0818995585505E-17,2.18));
#26898=CARTESIAN_POINT('Origin',(0.95,0.,2.35));
#26899=CARTESIAN_POINT('Origin',(0.935,0.,2.35));
#26900=CARTESIAN_POINT('',(0.935,-2.2655965784226E-17,2.165));
#26901=CARTESIAN_POINT('Origin',(0.7225,0.,2.35));
#26902=CARTESIAN_POINT('Origin',(0.5204,0.,2.35));
#26903=CARTESIAN_POINT('Origin',(0.4875,0.,2.35));
#26904=CARTESIAN_POINT('',(0.45,-1.53080849893419E-17,2.225));
#26905=CARTESIAN_POINT('Origin',(0.45,0.,2.35));
#26906=CARTESIAN_POINT('',(0.4875,-1.99005104861445E-17,2.1875));
#26907=CARTESIAN_POINT('Origin',(0.45,0.,2.35));
#31621=UNCERTAINTY_MEASURE_WITH_UNIT(LENGTH_MEASURE(0.001),#31639,
'DISTANCE_ACCURACY_VALUE',
'Maximum model space distance between geometric entities at asserted c
onnectivities');
#31625=UNCERTAINTY_MEASURE_WITH_UNIT(LENGTH_MEASURE(0.001),#31639,
'DISTANCE_ACCURACY_VALUE',
'Maximum model space distance between geometric entities at asserted c
onnectivities');
#31634=(
GEOMETRIC_REPRESENTATION_CONTEXT(3)
GLOBAL_UNCERTAINTY_ASSIGNED_CONTEXT((#31621))
GLOBAL_UNIT_ASSIGNED_CONTEXT((#31639,#31641,#31642))
REPRESENTATION_CONTEXT('','3D')
);
#31638=(
GEOMETRIC_REPRESENTATION_CONTEXT(3)
GLOBAL_UNCERTAINTY_ASSIGNED_CONTEXT((#31625))
GLOBAL_UNIT_ASSIGNED_CONTEXT((#31639,#31641,#31642))
REPRESENTATION_CONTEXT('','3D')
);
#31639=(
LENGTH_UNIT()
NAMED_UNIT(*)
SI_UNIT(.CENTI.,.METRE.)
);
#31641=(
NAMED_UNIT(*)
PLANE_ANGLE_UNIT()
SI_UNIT($,.RADIAN.)
);
#31642=(
NAMED_UNIT(*)
SI_UNIT($,.STERADIAN.)
SOLID_ANGLE_UNIT()
);
#31651=SHAPE_DEFINITION_REPRESENTATION(#31663,#31712);
#31663=PRODUCT_DEFINITION_SHAPE('',$,#31725);
#31712=SHAPE_REPRESENTATION('',(#13136),#31634);
#31716=PRODUCT_DEFINITION_CONTEXT('part definition',#31754,'design');
#31725=PRODUCT_DEFINITION('2026-10-22-02-42-23-427',
'08_ISO_4026_M4x5_Hex_Socket_Set_Screw_Flat_Point',#31737,#31716);
#31737=PRODUCT_DEFINITION_FORMATION('',$,#31764);
#31754=APPLICATION_CONTEXT(
'Core Data for Automotive Mechanical Design Process');
#31755=PRODUCT_CONTEXT('part definition',#31754,'mechanical');
#31764=PRODUCT('2026-10-22-02-42-23-427',
'08_ISO_4026_M4x5_Hex_Socket_Set_Screw_Flat_Point',$,(#31755));
#31831=COLOUR_RGB('Black',0.12,0.14,0.17);
#31832=FILL_AREA_STYLE_COLOUR('',#31831);
#31833=FILL_AREA_STYLE('',(#31832));
#31834=SURFACE_STYLE_FILL_AREA(#31833);
#31835=SURFACE_SIDE_STYLE('',(#31834));
#31836=SURFACE_STYLE_USAGE(.BOTH.,#31835);
#31837=PRESENTATION_STYLE_ASSIGNMENT((#31836));
ENDSEC;
END-ISO-10303-21;
